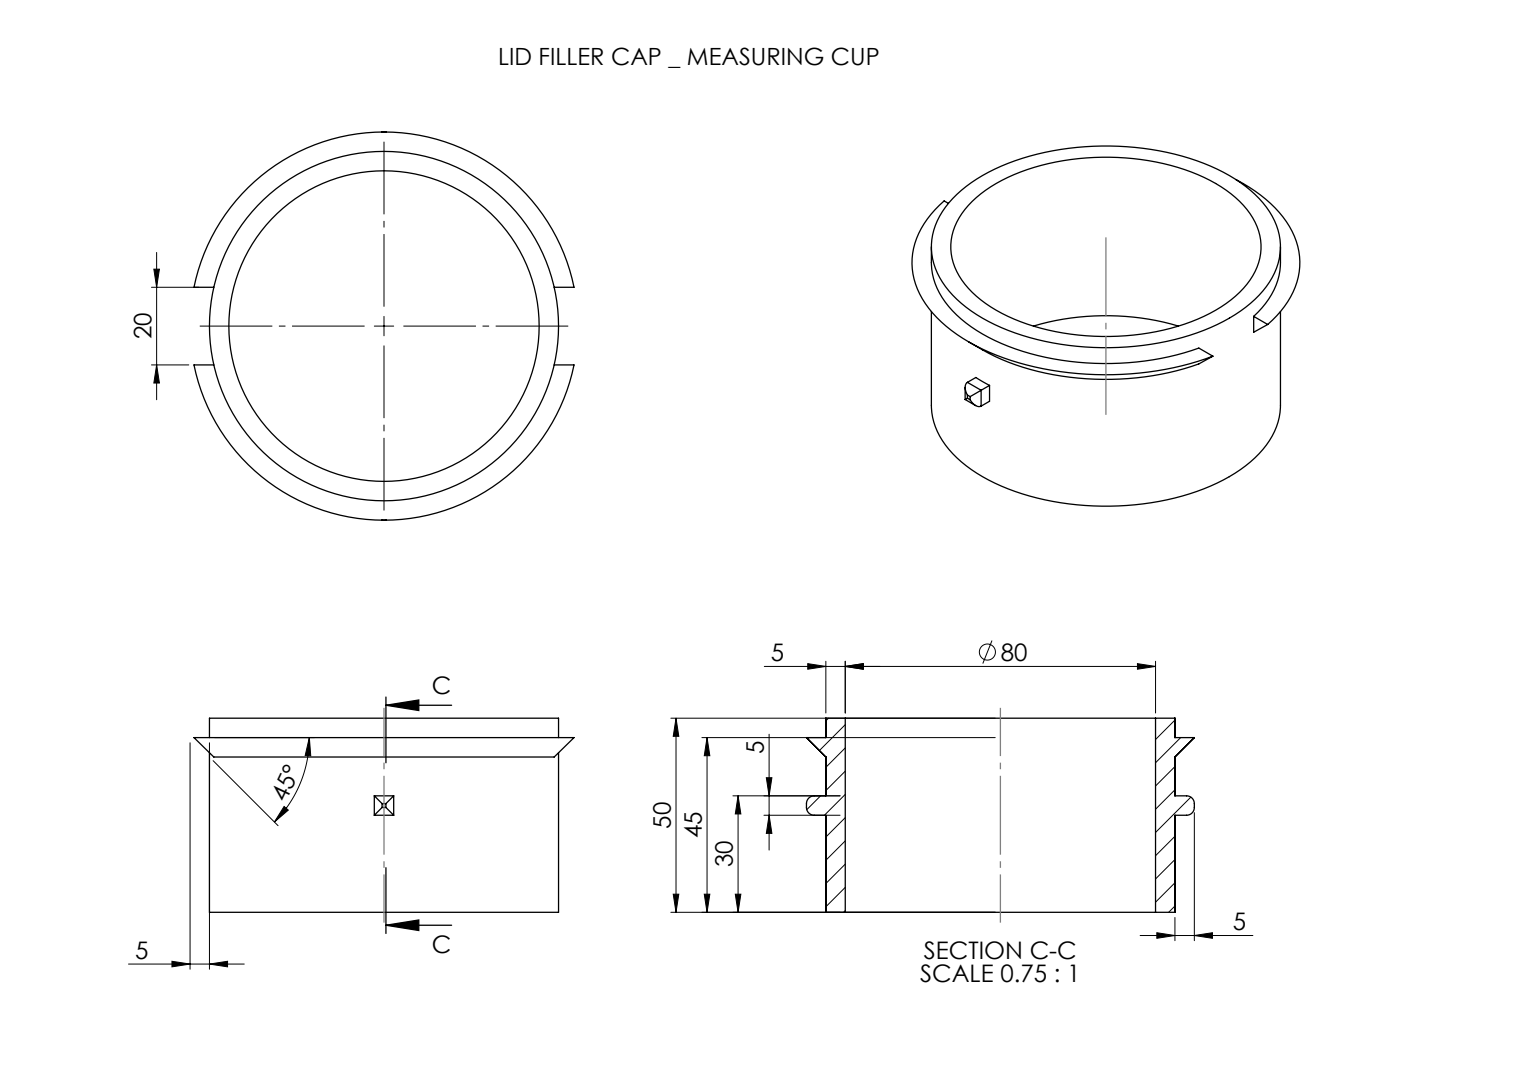
ISO-10303-21;
HEADER;
FILE_DESCRIPTION (('STEP AP214'),
    '1' );
FILE_NAME ('Lid Filler Cap _ Measuring Cup.step',
    '2026-10-09T15:02:13',
    ( '' ),
    ( '' ),
    'SwSTEP 2.0',
    'SolidWorks 2026',
    '' );
FILE_SCHEMA (( 'AUTOMOTIVE_DESIGN' ));
ENDSEC;

DATA;
#5=ORIENTED_EDGE ( 'NONE', *, *, #13422, .T. ) ;
#11=LINE ( 'NONE', #4013, #8670 ) ;
#38=CARTESIAN_POINT ( 'NONE',  ( -0.5000000000000000000, 247.0000000000000284, -49.99999999999999289 ) ) ;
#43=FACE_OUTER_BOUND ( 'NONE', #155, .T. ) ;
#49=( NAMED_UNIT ( * ) PLANE_ANGLE_UNIT ( ) SI_UNIT ( $, .RADIAN. ) );
#53=AXIS2_PLACEMENT_3D ( 'NONE', #15949, #12213, #9481 ) ;
#60=CARTESIAN_POINT ( 'NONE',  ( 48.98979485566356118, 261.9999999999999432, -10.00000000000000178 ) ) ;
#84=ADVANCED_FACE ( 'NONE', ( #9052 ), #9129, .T. ) ;
#99=EDGE_CURVE ( 'NONE', #10795, #16436, #8019, .T. ) ;
#105=CARTESIAN_POINT ( 'NONE',  ( 0.000000000000000000, 261.9999999999999432, 49.99999999999999289 ) ) ;
#115=CIRCLE ( 'NONE', #5192, 45.00000000000000000 ) ;
#121=AXIS2_PLACEMENT_3D ( 'NONE', #2630, #13768, #2460 ) ;
#129=( NAMED_UNIT ( * ) SI_UNIT ( $, .STERADIAN. ) SOLID_ANGLE_UNIT ( ) );
#140=AXIS2_PLACEMENT_3D ( 'NONE', #851, #930, #4703 ) ;
#149=LINE ( 'NONE', #6489, #8395 ) ;
#155=EDGE_LOOP ( 'NONE', ( #7318, #4198, #8287 ) ) ;
#161=PRESENTATION_STYLE_ASSIGNMENT (( #5178 ) ) ;
#164=CIRCLE ( 'NONE', #9467, 45.00000000000000000 ) ;
#227=DIRECTION ( 'NONE',  ( 0.000000000000000000, 0.000000000000000000, -1.000000000000000000 ) ) ;
#229=ORIENTED_EDGE ( 'NONE', *, *, #5927, .T. ) ;
#256=DIRECTION ( 'NONE',  ( 1.000000000000000000, -0.000000000000000000, 0.000000000000000000 ) ) ;
#260=CARTESIAN_POINT ( 'NONE',  ( 0.000000000000000000, 257.0000000000001137, 0.000000000000000000 ) ) ;
#277=LINE ( 'NONE', #1447, #969 ) ;
#314=DIRECTION ( 'NONE',  ( 0.000000000000000000, -1.000000000000000000, 0.000000000000000000 ) ) ;
#333=DIRECTION ( 'NONE',  ( 0.000000000000000000, 1.000000000000000000, 0.000000000000000000 ) ) ;
#350=DIRECTION ( 'NONE',  ( -0.000000000000000000, -1.000000000000000000, -0.000000000000000000 ) ) ;
#386=VECTOR ( 'NONE', #2589, 1000.000000000000000 ) ;
#407=EDGE_CURVE ( 'NONE', #5908, #14317, #4415, .T. ) ;
#409=CIRCLE ( 'NONE', #13951, 40.00000000000000000 ) ;
#441=EDGE_CURVE ( 'NONE', #7797, #13296, #9208, .T. ) ;
#442=AXIS2_PLACEMENT_3D ( 'NONE', #8820, #13970, #6598 ) ;
#469=ORIENTED_EDGE ( 'NONE', *, *, #407, .T. ) ;
#478=CARTESIAN_POINT ( 'NONE',  ( 0.5000000000000000000, 242.0000000000000284, -49.99999999999999289 ) ) ;
#516=CARTESIAN_POINT ( 'NONE',  ( 43.87482193696061472, 262.0000000000000000, -10.00000000000000000 ) ) ;
#573=CARTESIAN_POINT ( 'NONE',  ( 48.98979485566356118, 261.9999999999999432, -10.00000000000000178 ) ) ;
#590=EDGE_CURVE ( 'NONE', #9937, #12980, #2354, .T. ) ;
#613=ADVANCED_FACE ( 'NONE', ( #11344 ), #15222, .F. ) ;
#619=CIRCLE ( 'NONE', #8873, 45.00000000000000000 ) ;
#628=CARTESIAN_POINT ( 'NONE',  ( -43.87482193696060762, 257.0000000000001137, 10.00000000000000178 ) ) ;
#662=FACE_OUTER_BOUND ( 'NONE', #4298, .T. ) ;
#671=COLOUR_RGB ( '', 0.09019608, 0.27058824, 0.51372549) ;
#672=DIRECTION ( 'NONE',  ( 1.000000000000000000, 0.000000000000000000, -0.000000000000000000 ) ) ;
#693=VECTOR ( 'NONE', #7436, 1000.000000000000000 ) ;
#696=CIRCLE ( 'NONE', #10012, 45.00000000000000000 ) ;
#697=VECTOR ( 'NONE', #8943, 1000.000000000000000 ) ;
#709=AXIS2_PLACEMENT_3D ( 'NONE', #5217, #3952, #9026 ) ;
#716=EDGE_CURVE ( 'NONE', #9033, #5335, #1883, .T. ) ;
#740=ORIENTED_EDGE ( 'NONE', *, *, #6886, .T. ) ;
#751=CARTESIAN_POINT ( 'NONE',  ( -48.98979485566356828, 261.9999999999999432, -9.999999999999994671 ) ) ;
#799=ORIENTED_EDGE ( 'NONE', *, *, #441, .T. ) ;
#802=DIRECTION ( 'NONE',  ( 0.000000000000000000, 0.000000000000000000, 1.000000000000000000 ) ) ;
#814=ORIENTED_EDGE ( 'NONE', *, *, #8434, .F. ) ;
#826=EDGE_CURVE ( 'NONE', #11404, #10795, #164, .T. ) ;
#843=CARTESIAN_POINT ( 'NONE',  ( 0.000000000000000000, 267.0000000000000000, 0.000000000000000000 ) ) ;
#851=CARTESIAN_POINT ( 'NONE',  ( 0.000000000000000000, 247.0000000000000284, 0.000000000000000000 ) ) ;
#871=VERTEX_POINT ( 'NONE', #4096 ) ;
#930=DIRECTION ( 'NONE',  ( 0.000000000000000000, -1.000000000000000000, 0.000000000000000000 ) ) ;
#935=AXIS2_PLACEMENT_3D ( 'NONE', #14011, #3725, #13846 ) ;
#937=ORIENTED_EDGE ( 'NONE', *, *, #15743, .F. ) ;
#954=( GEOMETRIC_REPRESENTATION_CONTEXT ( 3 ) GLOBAL_UNCERTAINTY_ASSIGNED_CONTEXT ( ( #3259 ) ) GLOBAL_UNIT_ASSIGNED_CONTEXT ( ( #12888, #8987, #2830 ) ) REPRESENTATION_CONTEXT ( 'NONE', 'WORKASPACE' ) );
#958=DIRECTION ( 'NONE',  ( -0.000000000000000000, -1.000000000000000000, -0.000000000000000000 ) ) ;
#969=VECTOR ( 'NONE', #3869, 1000.000000000000000 ) ;
#1019=ADVANCED_FACE ( 'NONE', ( #14880 ), #4591, .T. ) ;
#1058=( BOUNDED_CURVE ( )  B_SPLINE_CURVE ( 3, ( #2059, #3401, #4566, #11138 ),
 .UNSPECIFIED., .F., .F. ) 
 B_SPLINE_CURVE_WITH_KNOTS ( ( 4, 4 ),
 ( 1.570796326794896780, 3.141592653589793116 ),
 .UNSPECIFIED. ) 
 CURVE ( )  GEOMETRIC_REPRESENTATION_ITEM ( )  RATIONAL_B_SPLINE_CURVE ( ( 1.000000000000000000, 0.8047378541243650485, 0.8047378541243650485, 1.000000000000000000 ) ) 
 REPRESENTATION_ITEM ( '' )  );
#1105=LINE ( 'NONE', #13997, #5701 ) ;
#1137=ORIENTED_EDGE ( 'NONE', *, *, #2862, .T. ) ;
#1152=DIRECTION ( 'NONE',  ( -0.000000000000000000, -1.000000000000000000, -0.000000000000000000 ) ) ;
#1159=VECTOR ( 'NONE', #14041, 1000.000000000000000 ) ;
#1167=DIRECTION ( 'NONE',  ( 0.000000000000000000, 0.000000000000000000, 1.000000000000000000 ) ) ;
#1174=CARTESIAN_POINT ( 'NONE',  ( 0.5000000000000000000, 244.0000000000000284, 49.99999999999999289 ) ) ;
#1176=DIRECTION ( 'NONE',  ( 1.000000000000000000, 0.000000000000000000, 0.000000000000000000 ) ) ;
#1191=DIRECTION ( 'NONE',  ( 1.000000000000000000, -0.000000000000000000, 0.000000000000000000 ) ) ;
#1216=( LENGTH_UNIT ( ) NAMED_UNIT ( * ) SI_UNIT ( .MILLI., .METRE. ) );
#1222=DIRECTION ( 'NONE',  ( -0.000000000000000000, 0.000000000000000000, -1.000000000000000000 ) ) ;
#1245=CARTESIAN_POINT ( 'NONE',  ( 2.500000000000000000, 242.0000000000000284, -47.99999999999999289 ) ) ;
#1256=DIRECTION ( 'NONE',  ( 0.000000000000000000, 0.000000000000000000, -1.000000000000000000 ) ) ;
#1301=FILL_AREA_STYLE ('',( #4995 ) ) ;
#1318=CARTESIAN_POINT ( 'NONE',  ( -2.500000000000000000, 242.0000000000000284, 40.00000000000000000 ) ) ;
#1323=ADVANCED_FACE ( 'NONE', ( #11720 ), #1654, .T. ) ;
#1328=VERTEX_POINT ( 'NONE', #9315 ) ;
#1335=PRODUCT_DEFINITION_SHAPE ( 'NONE', 'NONE',  #7215 ) ;
#1358=EDGE_CURVE ( 'NONE', #11111, #10385, #14441, .T. ) ;
#1359=DIRECTION ( 'NONE',  ( -0.000000000000000000, 1.000000000000000000, -0.000000000000000000 ) ) ;
#1364=PLANE ( 'NONE',  #709 ) ;
#1392=ORIENTED_EDGE ( 'NONE', *, *, #3028, .F. ) ;
#1394=CARTESIAN_POINT ( 'NONE',  ( 45.58196769024076644, 258.6644603543468861, -10.00000000000000178 ) ) ;
#1447=CARTESIAN_POINT ( 'NONE',  ( 0.000000000000000000, 242.0000000000000284, -47.99999999999999289 ) ) ;
#1454=CARTESIAN_POINT ( 'NONE',  ( -0.5000000000000000000, 244.0000000000000284, 49.99999999999999289 ) ) ;
#1465=ADVANCED_BREP_SHAPE_REPRESENTATION ( '', ( #14144, #15812 ), #5488 ) ;
#1490=CYLINDRICAL_SURFACE ( 'NONE', #7934, 40.00000000000000000 ) ;
#1491=CIRCLE ( 'NONE', #5765, 40.00000000000000000 ) ;
#1544=LINE ( 'NONE', #38, #15239 ) ;
#1555=CARTESIAN_POINT ( 'NONE',  ( 0.5000000000000000000, 245.0000000000000284, -49.99999999999999289 ) ) ;
#1581=ORIENTED_EDGE ( 'NONE', *, *, #8035, .T. ) ;
#1591=DIRECTION ( 'NONE',  ( 0.000000000000000000, -1.000000000000000000, 0.000000000000000000 ) ) ;
#1633=EDGE_CURVE ( 'NONE', #2064, #9033, #3918, .T. ) ;
#1645=LINE ( 'NONE', #10562, #16454 ) ;
#1654=CYLINDRICAL_SURFACE ( 'NONE', #4727, 2.000000000000001776 ) ;
#1661=ORIENTED_EDGE ( 'NONE', *, *, #2650, .F. ) ;
#1667=ORIENTED_EDGE ( 'NONE', *, *, #11380, .T. ) ;
#1686=DIRECTION ( 'NONE',  ( -1.000000000000000000, 0.000000000000000000, 0.000000000000000000 ) ) ;
#1700=VECTOR ( 'NONE', #10071, 1000.000000000000000 ) ;
#1704=EDGE_LOOP ( 'NONE', ( #4465, #8313, #12465, #9361 ) ) ;
#1759=CARTESIAN_POINT ( 'NONE',  ( -1.671572875253810153, 246.1715728752537871, -50.00000000000000000 ) ) ;
#1764=AXIS2_PLACEMENT_3D ( 'NONE', #2525, #15236, #15157 ) ;
#1805=ORIENTED_EDGE ( 'NONE', *, *, #3028, .T. ) ;
#1815=CARTESIAN_POINT ( 'NONE',  ( 0.000000000000000000, 242.0000000000000284, 0.000000000000000000 ) ) ;
#1825=CARTESIAN_POINT ( 'NONE',  ( -2.500000000000000000, 242.0000000000000284, -40.00000000000000000 ) ) ;
#1865=CARTESIAN_POINT ( 'NONE',  ( 0.000000000000000000, 217.0000000000000284, 0.000000000000000000 ) ) ;
#1883=( BOUNDED_CURVE ( )  B_SPLINE_CURVE ( 3, ( #11422, #10668, #1759, #14143 ),
 .UNSPECIFIED., .F., .F. ) 
 B_SPLINE_CURVE_WITH_KNOTS ( ( 4, 4 ),
 ( 3.141592653589793116, 4.712388980384689674 ),
 .UNSPECIFIED. ) 
 CURVE ( )  GEOMETRIC_REPRESENTATION_ITEM ( )  RATIONAL_B_SPLINE_CURVE ( ( 1.000000000000000000, 0.8047378541243649375, 0.8047378541243649375, 1.000000000000000000 ) ) 
 REPRESENTATION_ITEM ( '' )  );
#1911=CARTESIAN_POINT ( 'NONE',  ( 0.000000000000000000, 242.0000000000000284, 0.000000000000000000 ) ) ;
#1924=EDGE_CURVE ( 'NONE', #13942, #2064, #13776, .T. ) ;
#1931=DIRECTION ( 'NONE',  ( 0.000000000000000000, 1.000000000000000000, 0.000000000000000000 ) ) ;
#1943=CIRCLE ( 'NONE', #7794, 45.00000000000000000 ) ;
#1965=CARTESIAN_POINT ( 'NONE',  ( 0.000000000000000000, 261.9999999999999432, 0.000000000000000000 ) ) ;
#1968=CARTESIAN_POINT ( 'NONE',  ( 2.499999999999999556, 242.0000000000000284, -49.17157287525379417 ) ) ;
#1977=VERTEX_POINT ( 'NONE', #11381 ) ;
#1990=VECTOR ( 'NONE', #11855, 1000.000000000000000 ) ;
#2005=MECHANICAL_DESIGN_GEOMETRIC_PRESENTATION_REPRESENTATION('',(#13426),#15828);
#2028=MECHANICAL_DESIGN_GEOMETRIC_PRESENTATION_REPRESENTATION('',(#13447),#954);
#2054=CARTESIAN_POINT ( 'NONE',  ( -2.500000000000000000, 242.0000000000000284, 47.99999999999999289 ) ) ;
#2059=CARTESIAN_POINT ( 'NONE',  ( -0.5000000000000000000, 244.0000000000000284, 49.99999999999999289 ) ) ;
#2064=VERTEX_POINT ( 'NONE', #14677 ) ;
#2073=ORIENTED_EDGE ( 'NONE', *, *, #3686, .F. ) ;
#2110=ORIENTED_EDGE ( 'NONE', *, *, #14122, .T. ) ;
#2119=ORIENTED_EDGE ( 'NONE', *, *, #7947, .T. ) ;
#2122=ORIENTED_EDGE ( 'NONE', *, *, #13728, .T. ) ;
#2144=ORIENTED_EDGE ( 'NONE', *, *, #2862, .F. ) ;
#2154=CARTESIAN_POINT ( 'NONE',  ( -2.500000000000000000, 247.0000000000000284, 40.00000000000000000 ) ) ;
#2158=CARTESIAN_POINT ( 'NONE',  ( 0.000000000000000000, 0.000000000000000000, 0.000000000000000000 ) ) ;
#2161=DIRECTION ( 'NONE',  ( 0.000000000000000000, -1.000000000000000000, 0.000000000000000000 ) ) ;
#2189=AXIS2_PLACEMENT_3D ( 'NONE', #14664, #8362, #10630 ) ;
#2199=ORIENTED_EDGE ( 'NONE', *, *, #716, .T. ) ;
#2250=VERTEX_POINT ( 'NONE', #7390 ) ;
#2251=DIRECTION ( 'NONE',  ( -0.000000000000000000, -1.000000000000000000, -0.000000000000000000 ) ) ;
#2264=CARTESIAN_POINT ( 'NONE',  ( -0.5000000000000000000, 244.0000000000000284, -49.99999999999999289 ) ) ;
#2274=EDGE_CURVE ( 'NONE', #11502, #11404, #12970, .T. ) ;
#2295=EDGE_LOOP ( 'NONE', ( #3961, #2144 ) ) ;
#2305=CARTESIAN_POINT ( 'NONE',  ( 0.000000000000000000, 242.0000000000000284, 45.00000000000000000 ) ) ;
#2307=AXIS2_PLACEMENT_3D ( 'NONE', #15891, #14625, #3251 ) ;
#2308=CARTESIAN_POINT ( 'NONE',  ( 0.000000000000000000, 242.0000000000000284, 0.000000000000000000 ) ) ;
#2354=LINE ( 'NONE', #12578, #693 ) ;
#2380=FACE_OUTER_BOUND ( 'NONE', #2438, .T. ) ;
#2386=( LENGTH_UNIT ( ) NAMED_UNIT ( * ) SI_UNIT ( .MILLI., .METRE. ) );
#2408=CARTESIAN_POINT ( 'NONE',  ( -43.87482193696061472, 262.0000000000000000, 10.00000000000000178 ) ) ;
#2438=EDGE_LOOP ( 'NONE', ( #1392, #10459, #15571, #7122 ) ) ;
#2460=DIRECTION ( 'NONE',  ( 0.000000000000000000, 0.000000000000000000, 1.000000000000000000 ) ) ;
#2476=VERTEX_POINT ( 'NONE', #15965 ) ;
#2480=CARTESIAN_POINT ( 'NONE',  ( 4.898587196589413026E-15, 217.0000000000000284, -40.00000000000000000 ) ) ;
#2490=APPLICATION_CONTEXT ( 'automotive_design' ) ;
#2525=CARTESIAN_POINT ( 'NONE',  ( 0.000000000000000000, 262.0000000000000000, 0.000000000000000000 ) ) ;
#2530=DIRECTION ( 'NONE',  ( 0.000000000000000000, 0.000000000000000000, 1.000000000000000000 ) ) ;
#2565=ORIENTED_EDGE ( 'NONE', *, *, #99, .T. ) ;
#2570=AXIS2_PLACEMENT_3D ( 'NONE', #4839, #4664, #13620 ) ;
#2574=CARTESIAN_POINT ( 'NONE',  ( -43.87482193696061472, 257.0000000000001137, -10.00000000000000178 ) ) ;
#2589=DIRECTION ( 'NONE',  ( 1.000000000000000000, 0.000000000000000000, 0.000000000000000000 ) ) ;
#2600=DIRECTION ( 'NONE',  ( 0.000000000000000000, -1.000000000000000000, 0.000000000000000000 ) ) ;
#2626=ORIENTED_EDGE ( 'NONE', *, *, #7947, .F. ) ;
#2630=CARTESIAN_POINT ( 'NONE',  ( -0.5000000000000000000, 242.0000000000000284, 47.99999999999999289 ) ) ;
#2650=EDGE_CURVE ( 'NONE', #8967, #13787, #2656, .T. ) ;
#2653=CARTESIAN_POINT ( 'NONE',  ( 48.98979485566355407, 261.9999999999999432, 10.00000000000000178 ) ) ;
#2656=LINE ( 'NONE', #16381, #6623 ) ;
#2658=FACE_OUTER_BOUND ( 'NONE', #15932, .T. ) ;
#2661=ADVANCED_FACE ( 'NONE', ( #5016 ), #1490, .F. ) ;
#2673=DIRECTION ( 'NONE',  ( 0.000000000000000000, 0.000000000000000000, 1.000000000000000000 ) ) ;
#2688=ORIENTED_EDGE ( 'NONE', *, *, #3686, .T. ) ;
#2754=EDGE_CURVE ( 'NONE', #2831, #2833, #13123, .T. ) ;
#2773=CARTESIAN_POINT ( 'NONE',  ( 2.499999999999999556, 242.0000000000000284, 49.17157287525379417 ) ) ;
#2789=ORIENTED_EDGE ( 'NONE', *, *, #16426, .T. ) ;
#2801=CARTESIAN_POINT ( 'NONE',  ( 0.000000000000000000, 267.0000000000000000, 45.00000000000000000 ) ) ;
#2813=CARTESIAN_POINT ( 'NONE',  ( -2.500000000000000000, 242.0000000000000284, 40.00000000000000000 ) ) ;
#2817=AXIS2_PLACEMENT_3D ( 'NONE', #3359, #1931, #7024 ) ;
#2830=( NAMED_UNIT ( * ) SI_UNIT ( $, .STERADIAN. ) SOLID_ANGLE_UNIT ( ) );
#2831=VERTEX_POINT ( 'NONE', #4322 ) ;
#2833=VERTEX_POINT ( 'NONE', #2981 ) ;
#2862=EDGE_CURVE ( 'NONE', #8967, #11302, #6358, .T. ) ;
#2902=CARTESIAN_POINT ( 'NONE',  ( 0.000000000000000000, 257.0000000000001137, 0.000000000000000000 ) ) ;
#2918=ORIENTED_EDGE ( 'NONE', *, *, #4039, .T. ) ;
#2919=ORIENTED_EDGE ( 'NONE', *, *, #826, .T. ) ;
#2935=CYLINDRICAL_SURFACE ( 'NONE', #6732, 2.000000000000001776 ) ;
#2940=CARTESIAN_POINT ( 'NONE',  ( 2.500000000000000000, 242.0000000000000284, -49.99999999999999289 ) ) ;
#2959=DIRECTION ( 'NONE',  ( 0.000000000000000000, 0.000000000000000000, -1.000000000000000000 ) ) ;
#2960=CARTESIAN_POINT ( 'NONE',  ( -48.98979485566356118, 261.9999999999999432, 10.00000000000000178 ) ) ;
#2965=EDGE_CURVE ( 'NONE', #16436, #10385, #9551, .T. ) ;
#2981=CARTESIAN_POINT ( 'NONE',  ( -0.5000000000000000000, 245.0000000000000284, 49.99999999999999289 ) ) ;
#2990=CARTESIAN_POINT ( 'NONE',  ( -2.500000000000000000, 247.0000000000000284, -44.93050188902856945 ) ) ;
#3016=DIRECTION ( 'NONE',  ( -0.000000000000000000, -1.000000000000000000, -0.000000000000000000 ) ) ;
#3018=CARTESIAN_POINT ( 'NONE',  ( 0.5000000000000000000, 244.0000000000000284, 49.99999999999999289 ) ) ;
#3028=EDGE_CURVE ( 'NONE', #7197, #2833, #8692, .T. ) ;
#3031=VECTOR ( 'NONE', #12851, 1000.000000000000000 ) ;
#3035=CARTESIAN_POINT ( 'NONE',  ( -43.87482193696061472, 267.0000000000000000, -10.00000000000000178 ) ) ;
#3036=DIRECTION ( 'NONE',  ( -0.000000000000000000, 1.000000000000000000, -0.000000000000000000 ) ) ;
#3060=DIRECTION ( 'NONE',  ( -1.000000000000000000, -0.000000000000000000, -0.000000000000000000 ) ) ;
#3069=AXIS2_PLACEMENT_3D ( 'NONE', #3248, #6004, #16141 ) ;
#3076=VECTOR ( 'NONE', #2530, 1000.000000000000000 ) ;
#3157=VERTEX_POINT ( 'NONE', #2305 ) ;
#3183=CYLINDRICAL_SURFACE ( 'NONE', #4705, 2.000000000000001776 ) ;
#3239=DIRECTION ( 'NONE',  ( 1.000000000000000000, 0.000000000000000000, 0.000000000000000000 ) ) ;
#3248=CARTESIAN_POINT ( 'NONE',  ( 0.000000000000000000, 262.0000000000000000, 0.000000000000000000 ) ) ;
#3251=DIRECTION ( 'NONE',  ( 0.000000000000000000, 0.000000000000000000, 1.000000000000000000 ) ) ;
#3259=UNCERTAINTY_MEASURE_WITH_UNIT (LENGTH_MEASURE( 1.000000000000000082E-05 ), #12888, 'distance_accuracy_value', 'NONE');
#3309=DIRECTION ( 'NONE',  ( -0.000000000000000000, 1.000000000000000000, -0.000000000000000000 ) ) ;
#3322=FACE_OUTER_BOUND ( 'NONE', #12290, .T. ) ;
#3323=CARTESIAN_POINT ( 'NONE',  ( 0.000000000000000000, 217.0000000000000284, 0.000000000000000000 ) ) ;
#3325=LINE ( 'NONE', #5831, #7558 ) ;
#3341=ORIENTED_EDGE ( 'NONE', *, *, #9133, .T. ) ;
#3345=ORIENTED_EDGE ( 'NONE', *, *, #15831, .T. ) ;
#3347=CARTESIAN_POINT ( 'NONE',  ( 0.000000000000000000, 261.9999999999999432, 0.000000000000000000 ) ) ;
#3359=CARTESIAN_POINT ( 'NONE',  ( 0.000000000000000000, 257.0000000000001137, 0.000000000000000000 ) ) ;
#3373=EDGE_LOOP ( 'NONE', ( #1581, #13261, #7070, #7212 ) ) ;
#3400=CARTESIAN_POINT ( 'NONE',  ( -0.5000000000000000000, 245.0000000000000284, 49.99999999999999289 ) ) ;
#3401=CARTESIAN_POINT ( 'NONE',  ( -1.671572875253809487, 242.8284271247462129, 49.99999999999999289 ) ) ;
#3416=DIRECTION ( 'NONE',  ( -0.000000000000000000, 1.000000000000000000, -0.000000000000000000 ) ) ;
#3420=CARTESIAN_POINT ( 'NONE',  ( 2.500000000000000000, 247.0000000000000284, 47.99999999999999289 ) ) ;
#3427=CARTESIAN_POINT ( 'NONE',  ( 0.5000000000000000000, 245.0000000000000284, -49.99999999999999289 ) ) ;
#3456=VERTEX_POINT ( 'NONE', #2653 ) ;
#3471=ADVANCED_FACE ( 'NONE', ( #6329 ), #15195, .T. ) ;
#3487=DIRECTION ( 'NONE',  ( 1.000000000000000000, 0.000000000000000000, -0.000000000000000000 ) ) ;
#3496=CARTESIAN_POINT ( 'NONE',  ( 0.000000000000000000, 267.0000000000000000, 0.000000000000000000 ) ) ;
#3499=DIRECTION ( 'NONE',  ( -0.000000000000000000, -0.000000000000000000, -1.000000000000000000 ) ) ;
#3510=DIRECTION ( 'NONE',  ( 1.000000000000000000, 0.000000000000000000, 0.000000000000000000 ) ) ;
#3548=EDGE_LOOP ( 'NONE', ( #9663, #10724, #4831, #16342 ) ) ;
#3549=VECTOR ( 'NONE', #10900, 1000.000000000000000 ) ;
#3567=PLANE ( 'NONE',  #6457 ) ;
#3576=CYLINDRICAL_SURFACE ( 'NONE', #2570, 2.000000000000001776 ) ;
#3581=DIRECTION ( 'NONE',  ( 0.000000000000000000, 0.000000000000000000, 1.000000000000000000 ) ) ;
#3598=DIRECTION ( 'NONE',  ( 0.000000000000000000, -1.000000000000000000, 0.000000000000000000 ) ) ;
#3618=ORIENTED_EDGE ( 'NONE', *, *, #4491, .T. ) ;
#3625=CIRCLE ( 'NONE', #12915, 45.00000000000000000 ) ;
#3626=CIRCLE ( 'NONE', #5750, 45.00000000000000000 ) ;
#3684=ORIENTED_EDGE ( 'NONE', *, *, #7766, .F. ) ;
#3686=EDGE_CURVE ( 'NONE', #3456, #5700, #1645, .T. ) ;
#3687=EDGE_LOOP ( 'NONE', ( #8908, #8659, #937, #13226, #13943 ) ) ;
#3725=DIRECTION ( 'NONE',  ( 0.000000000000000000, 0.000000000000000000, -1.000000000000000000 ) ) ;
#3732=CARTESIAN_POINT ( 'NONE',  ( -2.500000000000000000, 242.0000000000000284, -40.00000000000000000 ) ) ;
#3758=VERTEX_POINT ( 'NONE', #4397 ) ;
#3781=ORIENTED_EDGE ( 'NONE', *, *, #8775, .T. ) ;
#3804=DIRECTION ( 'NONE',  ( 0.000000000000000000, 0.000000000000000000, -1.000000000000000000 ) ) ;
#3828=CARTESIAN_POINT ( 'NONE',  ( -45.00000000000000000, 262.0000000000000000, 10.00000000000000178 ) ) ;
#3829=DIRECTION ( 'NONE',  ( -0.000000000000000000, 1.000000000000000000, -0.000000000000000000 ) ) ;
#3830=CARTESIAN_POINT ( 'NONE',  ( 0.5000000000000000000, 247.0000000000000284, 49.99999999999999289 ) ) ;
#3839=CARTESIAN_POINT ( 'NONE',  ( 5.510910596163089556E-15, 217.0000000000000284, -45.00000000000000000 ) ) ;
#3869=DIRECTION ( 'NONE',  ( 1.000000000000000000, -0.000000000000000000, -0.000000000000000000 ) ) ;
#3878=ADVANCED_FACE ( 'NONE', ( #13205, #10801 ), #4318, .T. ) ;
#3883=PRODUCT_DEFINITION_FORMATION_WITH_SPECIFIED_SOURCE ( 'ANY', '', #8125, .NOT_KNOWN. ) ;
#3892=SURFACE_STYLE_FILL_AREA ( #1301 ) ;
#3896=AXIS2_PLACEMENT_3D ( 'NONE', #12478, #15963, #14700 ) ;
#3918=LINE ( 'NONE', #9070, #11352 ) ;
#3923=CARTESIAN_POINT ( 'NONE',  ( 45.58196769024076644, 258.6644603543468861, 10.00000000000000178 ) ) ;
#3927=CARTESIAN_POINT ( 'NONE',  ( 0.000000000000000000, 267.0000000000000000, 0.000000000000000000 ) ) ;
#3942=PRODUCT_DEFINITION_CONTEXT ( 'detailed design', #12378, 'design' ) ;
#3947=DIRECTION ( 'NONE',  ( 0.000000000000000000, 0.7071067811865362485, 0.7071067811865587860 ) ) ;
#3952=DIRECTION ( 'NONE',  ( -1.000000000000000000, 0.000000000000000000, 0.000000000000000000 ) ) ;
#3957=CARTESIAN_POINT ( 'NONE',  ( 2.500000000000000000, 245.0000000000000284, -49.99999999999999289 ) ) ;
#3961=ORIENTED_EDGE ( 'NONE', *, *, #4074, .F. ) ;
#4013=CARTESIAN_POINT ( 'NONE',  ( 0.000000000000000000, 247.0000000000000284, 47.99999999999999289 ) ) ;
#4039=EDGE_CURVE ( 'NONE', #16264, #14589, #15013, .T. ) ;
#4060=ADVANCED_FACE ( 'NONE', ( #15347 ), #12612, .T. ) ;
#4063=FACE_OUTER_BOUND ( 'NONE', #6879, .T. ) ;
#4073=DIRECTION ( 'NONE',  ( 0.000000000000000000, 0.000000000000000000, 1.000000000000000000 ) ) ;
#4074=EDGE_CURVE ( 'NONE', #11302, #8967, #409, .T. ) ;
#4094=CARTESIAN_POINT ( 'NONE',  ( -2.500000000000000000, 242.0000000000000284, 44.93050188902856945 ) ) ;
#4096=CARTESIAN_POINT ( 'NONE',  ( 2.500000000000000000, 242.0000000000000284, -44.93050188902856945 ) ) ;
#4163=VECTOR ( 'NONE', #3016, 1000.000000000000000 ) ;
#4170=CARTESIAN_POINT ( 'NONE',  ( 0.000000000000000000, 247.0000000000000284, 0.000000000000000000 ) ) ;
#4179=DIRECTION ( 'NONE',  ( -0.000000000000000000, -0.000000000000000000, -1.000000000000000000 ) ) ;
#4198=ORIENTED_EDGE ( 'NONE', *, *, #9133, .F. ) ;
#4221=FACE_OUTER_BOUND ( 'NONE', #8527, .T. ) ;
#4237=CARTESIAN_POINT ( 'NONE',  ( 0.5000000000000000000, 242.0000000000000284, 47.99999999999999289 ) ) ;
#4256=ORIENTED_EDGE ( 'NONE', *, *, #5027, .T. ) ;
#4258=DIRECTION ( 'NONE',  ( 1.000000000000000000, 0.000000000000000000, 0.000000000000000000 ) ) ;
#4280=CARTESIAN_POINT ( 'NONE',  ( 2.500000000000000000, 242.0000000000000284, 47.99999999999999289 ) ) ;
#4294=CARTESIAN_POINT ( 'NONE',  ( 2.500000000000000000, 244.0000000000000284, -49.99999999999999289 ) ) ;
#4298=EDGE_LOOP ( 'NONE', ( #16151, #2919, #2565, #11055, #3341 ) ) ;
#4301=ADVANCED_FACE ( 'NONE', ( #4221 ), #9288, .T. ) ;
#4312=VERTEX_POINT ( 'NONE', #2960 ) ;
#4315=DIRECTION ( 'NONE',  ( 0.000000000000000000, 0.000000000000000000, -1.000000000000000000 ) ) ;
#4318=PLANE ( 'NONE',  #14478 ) ;
#4322=CARTESIAN_POINT ( 'NONE',  ( 0.5000000000000000000, 245.0000000000000284, 49.99999999999999289 ) ) ;
#4324=DIRECTION ( 'NONE',  ( 0.000000000000000000, -1.000000000000000000, 0.000000000000000000 ) ) ;
#4326=DIRECTION ( 'NONE',  ( -1.000000000000000000, 0.000000000000000000, 0.000000000000000000 ) ) ;
#4329=CARTESIAN_POINT ( 'NONE',  ( 43.87482193696061472, 257.0000000000001137, 10.00000000000000178 ) ) ;
#4339=AXIS2_PLACEMENT_3D ( 'NONE', #12987, #1591, #6685 ) ;
#4358=CARTESIAN_POINT ( 'NONE',  ( -47.28673853953970507, 260.3313524089090265, 10.00000000000000178 ) ) ;
#4361=VECTOR ( 'NONE', #1152, 1000.000000000000000 ) ;
#4392=ORIENTED_EDGE ( 'NONE', *, *, #8165, .T. ) ;
#4393=ORIENTED_EDGE ( 'NONE', *, *, #2274, .F. ) ;
#4397=CARTESIAN_POINT ( 'NONE',  ( 5.510910596163089556E-15, 247.0000000000000284, -45.00000000000000000 ) ) ;
#4415=CIRCLE ( 'NONE', #2817, 45.00000000000000000 ) ;
#4437=AXIS2_PLACEMENT_3D ( 'NONE', #2308, #9629, #15018 ) ;
#4448=VECTOR ( 'NONE', #1191, 1000.000000000000000 ) ;
#4462=EDGE_LOOP ( 'NONE', ( #2789, #14991, #12051, #16393, #13020, #2688 ) ) ;
#4465=ORIENTED_EDGE ( 'NONE', *, *, #7682, .T. ) ;
#4481=ORIENTED_EDGE ( 'NONE', *, *, #15955, .F. ) ;
#4491=EDGE_CURVE ( 'NONE', #12980, #7494, #8769, .T. ) ;
#4496=ORIENTED_EDGE ( 'NONE', *, *, #16426, .F. ) ;
#4518=AXIS2_PLACEMENT_3D ( 'NONE', #1965, #5812, #4565 ) ;
#4530=CYLINDRICAL_SURFACE ( 'NONE', #7074, 2.000000000000001776 ) ;
#4565=DIRECTION ( 'NONE',  ( 0.000000000000000000, 0.000000000000000000, -1.000000000000000000 ) ) ;
#4566=CARTESIAN_POINT ( 'NONE',  ( -2.499999999999999556, 242.0000000000000284, 49.17157287525379417 ) ) ;
#4583=FACE_OUTER_BOUND ( 'NONE', #6617, .T. ) ;
#4591=PLANE ( 'NONE',  #10558 ) ;
#4597=CARTESIAN_POINT ( 'NONE',  ( -2.500000000000000000, 217.0000000000000284, -44.93050188902856945 ) ) ;
#4635=PLANE ( 'NONE',  #2189 ) ;
#4662=ORIENTED_EDGE ( 'NONE', *, *, #8269, .F. ) ;
#4664=DIRECTION ( 'NONE',  ( 0.000000000000000000, 1.000000000000000000, 0.000000000000000000 ) ) ;
#4673=VECTOR ( 'NONE', #5576, 1000.000000000000000 ) ;
#4698=CLOSED_SHELL ( 'NONE', ( #6928, #10284, #4060, #14884, #6739, #4301, #3878, #8847, #2661, #10035, #10518, #14607, #11167, #11202, #1019, #613, #6021, #12253, #3471, #13850, #5707, #11911, #1323, #84, #15145, #9635, #11125, #4837, #12291, #9610, #10662, #9826, #11496 ) ) ;
#4703=DIRECTION ( 'NONE',  ( 0.000000000000000000, 0.000000000000000000, -1.000000000000000000 ) ) ;
#4705=AXIS2_PLACEMENT_3D ( 'NONE', #15903, #10676, #15575 ) ;
#4727=AXIS2_PLACEMENT_3D ( 'NONE', #11884, #4326, #4073 ) ;
#4756=ORIENTED_EDGE ( 'NONE', *, *, #15914, .F. ) ;
#4774=DIRECTION ( 'NONE',  ( 0.000000000000000000, 0.000000000000000000, 1.000000000000000000 ) ) ;
#4799=ORIENTED_EDGE ( 'NONE', *, *, #9262, .F. ) ;
#4802=ORIENTED_EDGE ( 'NONE', *, *, #14156, .F. ) ;
#4831=ORIENTED_EDGE ( 'NONE', *, *, #1924, .F. ) ;
#4837=ADVANCED_FACE ( 'NONE', ( #15906 ), #4530, .T. ) ;
#4839=CARTESIAN_POINT ( 'NONE',  ( 0.5000000000000000000, 242.0000000000000284, -47.99999999999999289 ) ) ;
#4909=SHAPE_REPRESENTATION_RELATIONSHIP ( 'NONE' , 'NONE' ,  #5560, #1465 ) ;
#4933=DIRECTION ( 'NONE',  ( 0.000000000000000000, 0.000000000000000000, 1.000000000000000000 ) ) ;
#4936=AXIS2_PLACEMENT_3D ( 'NONE', #13137, #15707, #4258 ) ;
#4943=ORIENTED_EDGE ( 'NONE', *, *, #5027, .F. ) ;
#4965=EDGE_LOOP ( 'NONE', ( #740, #12195, #4756 ) ) ;
#4995=FILL_AREA_STYLE_COLOUR ( '', #671 ) ;
#5015=LINE ( 'NONE', #1318, #7534 ) ;
#5016=FACE_OUTER_BOUND ( 'NONE', #5518, .T. ) ;
#5027=EDGE_CURVE ( 'NONE', #7197, #7494, #11, .T. ) ;
#5042=CARTESIAN_POINT ( 'NONE',  ( 0.000000000000000000, 247.0000000000000284, 0.000000000000000000 ) ) ;
#5089=CARTESIAN_POINT ( 'NONE',  ( -2.500000000000000000, 242.0000000000000284, 49.99999999999999289 ) ) ;
#5092=DIRECTION ( 'NONE',  ( 0.000000000000000000, 0.000000000000000000, 1.000000000000000000 ) ) ;
#5095=LINE ( 'NONE', #15200, #4361 ) ;
#5157=EDGE_LOOP ( 'NONE', ( #8102, #10104, #5992, #5888 ) ) ;
#5165=CARTESIAN_POINT ( 'NONE',  ( 47.28673853953970507, 260.3313524089090265, -10.00000000000000178 ) ) ;
#5172=CARTESIAN_POINT ( 'NONE',  ( 0.000000000000000000, 217.0000000000000284, 0.000000000000000000 ) ) ;
#5178=SURFACE_STYLE_USAGE ( .BOTH. , #7737 ) ;
#5183=LINE ( 'NONE', #8993, #386 ) ;
#5192=AXIS2_PLACEMENT_3D ( 'NONE', #3323, #14950, #3239 ) ;
#5217=CARTESIAN_POINT ( 'NONE',  ( 2.500000000000000000, 242.0000000000000284, 40.00000000000000000 ) ) ;
#5223=( BOUNDED_CURVE ( )  B_SPLINE_CURVE ( 3, ( #13453, #12036, #1968, #9557 ),
 .UNSPECIFIED., .F., .T. ) 
 B_SPLINE_CURVE_WITH_KNOTS ( ( 4, 4 ),
 ( 1.570796326794896780, 3.141592653589793116 ),
 .UNSPECIFIED. ) 
 CURVE ( )  GEOMETRIC_REPRESENTATION_ITEM ( )  RATIONAL_B_SPLINE_CURVE ( ( 1.000000000000000000, 0.8047378541243650485, 0.8047378541243650485, 1.000000000000000000 ) ) 
 REPRESENTATION_ITEM ( '' )  );
#5228=EDGE_LOOP ( 'NONE', ( #799, #9813, #2199, #4662 ) ) ;
#5237=DIRECTION ( 'NONE',  ( -0.000000000000000000, 1.000000000000000000, -0.000000000000000000 ) ) ;
#5295=ORIENTED_EDGE ( 'NONE', *, *, #10543, .T. ) ;
#5335=VERTEX_POINT ( 'NONE', #8809 ) ;
#5357=CARTESIAN_POINT ( 'NONE',  ( 0.000000000000000000, 267.0000000000000000, 0.000000000000000000 ) ) ;
#5413=CARTESIAN_POINT ( 'NONE',  ( -2.500000000000000000, 245.0000000000000284, 49.99999999999999289 ) ) ;
#5421=DIRECTION ( 'NONE',  ( 0.000000000000000000, 0.000000000000000000, -1.000000000000000000 ) ) ;
#5449=FACE_OUTER_BOUND ( 'NONE', #5157, .T. ) ;
#5468=VERTEX_POINT ( 'NONE', #2408 ) ;
#5488=( GEOMETRIC_REPRESENTATION_CONTEXT ( 3 ) GLOBAL_UNCERTAINTY_ASSIGNED_CONTEXT ( ( #12067 ) ) GLOBAL_UNIT_ASSIGNED_CONTEXT ( ( #2386, #13690, #16444 ) ) REPRESENTATION_CONTEXT ( 'NONE', 'WORKASPACE' ) );
#5498=CIRCLE ( 'NONE', #14753, 40.00000000000000000 ) ;
#5518=EDGE_LOOP ( 'NONE', ( #1661, #1137, #2119, #5851 ) ) ;
#5529=AXIS2_PLACEMENT_3D ( 'NONE', #2813, #5575, #11635 ) ;
#5540=LINE ( 'NONE', #4280, #4163 ) ;
#5560=SHAPE_REPRESENTATION ( 'Lid Filler Cap _ Measuring Cup', ( #15812 ), #5488 ) ;
#5564=DIRECTION ( 'NONE',  ( -1.000000000000000000, 0.000000000000000000, 0.000000000000000000 ) ) ;
#5575=DIRECTION ( 'NONE',  ( -1.000000000000000000, 0.000000000000000000, 0.000000000000000000 ) ) ;
#5576=DIRECTION ( 'NONE',  ( -0.000000000000000000, -1.000000000000000000, -0.000000000000000000 ) ) ;
#5577=DIRECTION ( 'NONE',  ( 0.000000000000000000, -0.000000000000000000, -1.000000000000000000 ) ) ;
#5643=FACE_OUTER_BOUND ( 'NONE', #3373, .T. ) ;
#5700=VERTEX_POINT ( 'NONE', #10781 ) ;
#5701=VECTOR ( 'NONE', #1359, 1000.000000000000000 ) ;
#5702=DIRECTION ( 'NONE',  ( -1.000000000000000000, 0.000000000000000000, 0.000000000000000000 ) ) ;
#5707=ADVANCED_FACE ( 'NONE', ( #6725 ), #10545, .T. ) ;
#5721=ORIENTED_EDGE ( 'NONE', *, *, #2754, .T. ) ;
#5725=CARTESIAN_POINT ( 'NONE',  ( 2.500000000000000000, 242.0000000000000284, -47.99999999999999289 ) ) ;
#5750=AXIS2_PLACEMENT_3D ( 'NONE', #14715, #8498, #6104 ) ;
#5753=CARTESIAN_POINT ( 'NONE',  ( -2.500000000000000000, 242.0000000000000284, -47.99999999999999289 ) ) ;
#5765=AXIS2_PLACEMENT_3D ( 'NONE', #843, #3598, #10002 ) ;
#5773=VECTOR ( 'NONE', #14163, 1000.000000000000000 ) ;
#5807=DIRECTION ( 'NONE',  ( -1.000000000000000000, 0.000000000000000000, 0.000000000000000000 ) ) ;
#5812=DIRECTION ( 'NONE',  ( -0.000000000000000000, -1.000000000000000000, -0.000000000000000000 ) ) ;
#5815=CARTESIAN_POINT ( 'NONE',  ( -2.500000000000000000, 247.0000000000000284, 47.99999999999999289 ) ) ;
#5831=CARTESIAN_POINT ( 'NONE',  ( 0.000000000000000000, 217.0000000000000284, 40.00000000000000000 ) ) ;
#5834=CARTESIAN_POINT ( 'NONE',  ( 0.000000000000000000, 261.9999999999999432, 0.000000000000000000 ) ) ;
#5835=LINE ( 'NONE', #8239, #3549 ) ;
#5851=ORIENTED_EDGE ( 'NONE', *, *, #13222, .F. ) ;
#5886=EDGE_LOOP ( 'NONE', ( #10870, #11725, #2073 ) ) ;
#5888=ORIENTED_EDGE ( 'NONE', *, *, #5959, .F. ) ;
#5908=VERTEX_POINT ( 'NONE', #7772 ) ;
#5916=EDGE_CURVE ( 'NONE', #13296, #9545, #277, .T. ) ;
#5927=EDGE_CURVE ( 'NONE', #2250, #10795, #10192, .T. ) ;
#5959=EDGE_CURVE ( 'NONE', #8386, #6499, #10353, .T. ) ;
#5978=CARTESIAN_POINT ( 'NONE',  ( -1.671572875253810153, 246.1715728752537871, 50.00000000000000000 ) ) ;
#5987=EDGE_CURVE ( 'NONE', #3758, #11404, #11514, .T. ) ;
#5992=ORIENTED_EDGE ( 'NONE', *, *, #8035, .F. ) ;
#6000=CARTESIAN_POINT ( 'NONE',  ( 0.000000000000000000, 267.0000000000000000, 0.000000000000000000 ) ) ;
#6004=DIRECTION ( 'NONE',  ( -0.000000000000000000, -1.000000000000000000, -0.000000000000000000 ) ) ;
#6013=ORIENTED_EDGE ( 'NONE', *, *, #441, .F. ) ;
#6017=ORIENTED_EDGE ( 'NONE', *, *, #13167, .F. ) ;
#6021=ADVANCED_FACE ( 'NONE', ( #12765 ), #1364, .F. ) ;
#6030=AXIS2_PLACEMENT_3D ( 'NONE', #6699, #672, #13081 ) ;
#6089=CARTESIAN_POINT ( 'NONE',  ( 0.5000000000000000000, 245.0000000000000284, 49.99999999999999289 ) ) ;
#6099=DIRECTION ( 'NONE',  ( 0.000000000000000000, 1.000000000000000000, 0.000000000000000000 ) ) ;
#6104=DIRECTION ( 'NONE',  ( 0.000000000000000000, 0.000000000000000000, -1.000000000000000000 ) ) ;
#6136=ORIENTED_EDGE ( 'NONE', *, *, #11659, .F. ) ;
#6181=FACE_OUTER_BOUND ( 'NONE', #4462, .T. ) ;
#6218=EDGE_CURVE ( 'NONE', #14271, #3758, #11571, .T. ) ;
#6223=AXIS2_PLACEMENT_3D ( 'NONE', #8810, #10148, #4933 ) ;
#6233=VECTOR ( 'NONE', #3499, 1000.000000000000000 ) ;
#6259=CARTESIAN_POINT ( 'NONE',  ( 48.98979485566355407, 261.9999999999999432, 10.00000000000000178 ) ) ;
#6280=ORIENTED_EDGE ( 'NONE', *, *, #11036, .F. ) ;
#6305=CARTESIAN_POINT ( 'NONE',  ( 0.000000000000000000, 217.0000000000000284, 0.000000000000000000 ) ) ;
#6329=FACE_OUTER_BOUND ( 'NONE', #10890, .T. ) ;
#6348=CARTESIAN_POINT ( 'NONE',  ( 0.000000000000000000, 217.0000000000000284, 0.000000000000000000 ) ) ;
#6358=CIRCLE ( 'NONE', #15633, 40.00000000000000000 ) ;
#6392=SURFACE_SIDE_STYLE ('',( #3892 ) ) ;
#6415=CARTESIAN_POINT ( 'NONE',  ( 0.000000000000000000, 242.0000000000000284, 0.000000000000000000 ) ) ;
#6452=CARTESIAN_POINT ( 'NONE',  ( 2.500000000000000000, 247.0000000000000284, 40.00000000000000000 ) ) ;
#6457=AXIS2_PLACEMENT_3D ( 'NONE', #3732, #3487, #1222 ) ;
#6479=DIRECTION ( 'NONE',  ( 1.000000000000000000, 0.000000000000000000, 0.000000000000000000 ) ) ;
#6487=DIRECTION ( 'NONE',  ( -0.000000000000000000, 0.000000000000000000, 1.000000000000000000 ) ) ;
#6489=CARTESIAN_POINT ( 'NONE',  ( -2.500000000000000000, 242.0000000000000284, -47.99999999999999289 ) ) ;
#6499=VERTEX_POINT ( 'NONE', #1174 ) ;
#6521=B_SPLINE_CURVE_WITH_KNOTS ( 'NONE', 3,
 ( #60, #5165, #1394, #15275 ),
 .UNSPECIFIED., .F., .F.,
 ( 4, 4 ),
 ( 0.01002676606614814371, 0.01717959331248046853 ),
 .UNSPECIFIED. ) ;
#6523=AXIS2_PLACEMENT_3D ( 'NONE', #3035, #2959, #8106 ) ;
#6571=VERTEX_POINT ( 'NONE', #4094 ) ;
#6572=CARTESIAN_POINT ( 'NONE',  ( -47.28673853953969797, 260.3313524089090265, -10.00000000000000178 ) ) ;
#6589=DIRECTION ( 'NONE',  ( 1.000000000000000000, 0.000000000000000000, 0.000000000000000000 ) ) ;
#6592=DIRECTION ( 'NONE',  ( 0.000000000000000000, -1.000000000000000000, 0.000000000000000000 ) ) ;
#6598=DIRECTION ( 'NONE',  ( 1.000000000000000000, 0.000000000000000000, -0.000000000000000000 ) ) ;
#6601=DIRECTION ( 'NONE',  ( -0.000000000000000000, 1.000000000000000000, -0.000000000000000000 ) ) ;
#6617=EDGE_LOOP ( 'NONE', ( #3684, #469, #9794, #12943 ) ) ;
#6618=LINE ( 'NONE', #7604, #7345 ) ;
#6623=VECTOR ( 'NONE', #12881, 1000.000000000000000 ) ;
#6657=VERTEX_POINT ( 'NONE', #3427 ) ;
#6660=LINE ( 'NONE', #14280, #4673 ) ;
#6683=DIRECTION ( 'NONE',  ( -0.000000000000000000, 1.000000000000000000, -0.000000000000000000 ) ) ;
#6685=DIRECTION ( 'NONE',  ( 0.000000000000000000, 0.000000000000000000, -1.000000000000000000 ) ) ;
#6696=ORIENTED_EDGE ( 'NONE', *, *, #4491, .F. ) ;
#6699=CARTESIAN_POINT ( 'NONE',  ( 2.500000000000000000, 242.0000000000000284, -40.00000000000000000 ) ) ;
#6716=ORIENTED_EDGE ( 'NONE', *, *, #14306, .T. ) ;
#6718=LINE ( 'NONE', #7950, #1990 ) ;
#6725=FACE_OUTER_BOUND ( 'NONE', #10344, .T. ) ;
#6727=PRODUCT_CONTEXT ( 'NONE', #2490, 'mechanical' ) ;
#6732=AXIS2_PLACEMENT_3D ( 'NONE', #8002, #13076, #10594 ) ;
#6739=ADVANCED_FACE ( 'NONE', ( #662 ), #14593, .T. ) ;
#6785=VECTOR ( 'NONE', #3416, 1000.000000000000000 ) ;
#6809=SHAPE_DEFINITION_REPRESENTATION ( #1335, #5560 ) ;
#6825=AXIS2_PLACEMENT_3D ( 'NONE', #12870, #6479, #227 ) ;
#6861=DIRECTION ( 'NONE',  ( 0.000000000000000000, 0.000000000000000000, 1.000000000000000000 ) ) ;
#6879=EDGE_LOOP ( 'NONE', ( #15611, #14191, #13747, #11446 ) ) ;
#6886=EDGE_CURVE ( 'NONE', #5468, #9544, #5095, .T. ) ;
#6907=DIRECTION ( 'NONE',  ( 0.000000000000000000, 0.000000000000000000, -1.000000000000000000 ) ) ;
#6912=ORIENTED_EDGE ( 'NONE', *, *, #8796, .T. ) ;
#6913=( BOUNDED_CURVE ( )  B_SPLINE_CURVE ( 3, ( #3018, #13163, #2773, #10516 ),
 .UNSPECIFIED., .F., .F. ) 
 B_SPLINE_CURVE_WITH_KNOTS ( ( 4, 4 ),
 ( 1.570796326794896780, 3.141592653589793116 ),
 .UNSPECIFIED. ) 
 CURVE ( )  GEOMETRIC_REPRESENTATION_ITEM ( )  RATIONAL_B_SPLINE_CURVE ( ( 1.000000000000000000, 0.8047378541243650485, 0.8047378541243650485, 1.000000000000000000 ) ) 
 REPRESENTATION_ITEM ( '' )  );
#6928=ADVANCED_FACE ( 'NONE', ( #2658 ), #10467, .T. ) ;
#6936=EDGE_CURVE ( 'NONE', #6499, #2831, #7567, .T. ) ;
#6940=CARTESIAN_POINT ( 'NONE',  ( -48.98979485566356118, 261.9999999999999432, 10.00000000000000178 ) ) ;
#6967=EDGE_CURVE ( 'NONE', #14589, #7197, #13715, .T. ) ;
#6979=DIRECTION ( 'NONE',  ( -0.000000000000000000, -1.000000000000000000, -0.000000000000000000 ) ) ;
#6985=ORIENTED_EDGE ( 'NONE', *, *, #15743, .T. ) ;
#7010=LINE ( 'NONE', #4597, #10703 ) ;
#7015=DIRECTION ( 'NONE',  ( -0.000000000000000000, 0.000000000000000000, -1.000000000000000000 ) ) ;
#7024=DIRECTION ( 'NONE',  ( 0.000000000000000000, 0.000000000000000000, 1.000000000000000000 ) ) ;
#7041=CIRCLE ( 'NONE', #4936, 45.00000000000000000 ) ;
#7058=EDGE_CURVE ( 'NONE', #2476, #871, #619, .T. ) ;
#7063=VECTOR ( 'NONE', #14789, 1000.000000000000000 ) ;
#7070=ORIENTED_EDGE ( 'NONE', *, *, #10581, .T. ) ;
#7074=AXIS2_PLACEMENT_3D ( 'NONE', #9593, #14640, #9764 ) ;
#7075=AXIS2_PLACEMENT_3D ( 'NONE', #15062, #9668, #14808 ) ;
#7083=LINE ( 'NONE', #7327, #11315 ) ;
#7084=DIRECTION ( 'NONE',  ( 0.000000000000000000, -1.000000000000000000, 0.000000000000000000 ) ) ;
#7122=ORIENTED_EDGE ( 'NONE', *, *, #9357, .F. ) ;
#7154=EDGE_LOOP ( 'NONE', ( #1667, #9461 ) ) ;
#7163=ORIENTED_EDGE ( 'NONE', *, *, #7330, .F. ) ;
#7182=CARTESIAN_POINT ( 'NONE',  ( 2.500000000000000000, 247.0000000000000284, 44.93050188902856945 ) ) ;
#7197=VERTEX_POINT ( 'NONE', #5815 ) ;
#7212=ORIENTED_EDGE ( 'NONE', *, *, #6936, .F. ) ;
#7215=PRODUCT_DEFINITION ( 'UNKNOWN', '', #3883, #3942 ) ;
#7237=DIRECTION ( 'NONE',  ( 0.000000000000000000, -0.000000000000000000, -1.000000000000000000 ) ) ;
#7244=LINE ( 'NONE', #8317, #8862 ) ;
#7274=CARTESIAN_POINT ( 'NONE',  ( -1.671572875253809487, 242.8284271247462129, -50.00000000000000000 ) ) ;
#7304=VECTOR ( 'NONE', #4179, 1000.000000000000000 ) ;
#7318=ORIENTED_EDGE ( 'NONE', *, *, #11093, .T. ) ;
#7327=CARTESIAN_POINT ( 'NONE',  ( -2.500000000000000000, 217.0000000000000284, 44.93050188902856945 ) ) ;
#7330=EDGE_CURVE ( 'NONE', #9682, #9545, #5223, .T. ) ;
#7345=VECTOR ( 'NONE', #350, 1000.000000000000000 ) ;
#7358=AXIS2_PLACEMENT_3D ( 'NONE', #4170, #6592, #5421 ) ;
#7368=VECTOR ( 'NONE', #6589, 1000.000000000000000 ) ;
#7390=CARTESIAN_POINT ( 'NONE',  ( -43.87482193696061472, 262.0000000000000000, -10.00000000000000178 ) ) ;
#7421=ORIENTED_EDGE ( 'NONE', *, *, #11209, .T. ) ;
#7426=DIRECTION ( 'NONE',  ( 0.000000000000000000, 1.000000000000000000, 0.000000000000000000 ) ) ;
#7436=DIRECTION ( 'NONE',  ( -0.000000000000000000, 1.000000000000000000, -0.000000000000000000 ) ) ;
#7494=VERTEX_POINT ( 'NONE', #8964 ) ;
#7500=DIRECTION ( 'NONE',  ( 0.000000000000000000, -1.000000000000000000, -0.000000000000000000 ) ) ;
#7534=VECTOR ( 'NONE', #5092, 1000.000000000000000 ) ;
#7556=ORIENTED_EDGE ( 'NONE', *, *, #13811, .F. ) ;
#7558=VECTOR ( 'NONE', #10603, 1000.000000000000000 ) ;
#7567=LINE ( 'NONE', #3830, #1159 ) ;
#7582=CYLINDRICAL_SURFACE ( 'NONE', #8122, 40.00000000000000000 ) ;
#7593=AXIS2_PLACEMENT_3D ( 'NONE', #11374, #5237, #7706 ) ;
#7604=CARTESIAN_POINT ( 'NONE',  ( 43.87482193696061472, 267.0000000000000000, -10.00000000000000000 ) ) ;
#7621=LINE ( 'NONE', #3957, #3031 ) ;
#7640=VERTEX_POINT ( 'NONE', #14268 ) ;
#7682=EDGE_CURVE ( 'NONE', #2064, #6657, #13684, .T. ) ;
#7706=DIRECTION ( 'NONE',  ( 0.000000000000000000, 0.000000000000000000, 1.000000000000000000 ) ) ;
#7715=ORIENTED_EDGE ( 'NONE', *, *, #7682, .F. ) ;
#7718=ORIENTED_EDGE ( 'NONE', *, *, #11659, .T. ) ;
#7722=ORIENTED_EDGE ( 'NONE', *, *, #6936, .T. ) ;
#7737=SURFACE_SIDE_STYLE ('',( #15293 ) ) ;
#7742=DIRECTION ( 'NONE',  ( 0.000000000000000000, 0.000000000000000000, 1.000000000000000000 ) ) ;
#7766=EDGE_CURVE ( 'NONE', #5908, #1328, #10029, .T. ) ;
#7772=CARTESIAN_POINT ( 'NONE',  ( 0.000000000000000000, 257.0000000000001137, 45.00000000000000000 ) ) ;
#7778=EDGE_CURVE ( 'NONE', #871, #13942, #1105, .T. ) ;
#7794=AXIS2_PLACEMENT_3D ( 'NONE', #6000, #7084, #11070 ) ;
#7797=VERTEX_POINT ( 'NONE', #12592 ) ;
#7821=PLANE ( 'NONE',  #442 ) ;
#7844=ORIENTED_EDGE ( 'NONE', *, *, #7330, .T. ) ;
#7875=CARTESIAN_POINT ( 'NONE',  ( 1.671572875253809487, 246.1715728752537871, -50.00000000000000000 ) ) ;
#7908=LINE ( 'NONE', #10163, #13692 ) ;
#7923=AXIS2_PLACEMENT_3D ( 'NONE', #10206, #11214, #10046 ) ;
#7934=AXIS2_PLACEMENT_3D ( 'NONE', #5172, #3829, #10229 ) ;
#7947=EDGE_CURVE ( 'NONE', #11302, #10383, #3325, .T. ) ;
#7950=CARTESIAN_POINT ( 'NONE',  ( 2.500000000000000000, 242.0000000000000284, 40.00000000000000000 ) ) ;
#7965=EDGE_LOOP ( 'NONE', ( #9323, #2918, #4481, #7718, #2110 ) ) ;
#8002=CARTESIAN_POINT ( 'NONE',  ( -0.5000000000000000000, 242.0000000000000284, -47.99999999999999289 ) ) ;
#8019=B_SPLINE_CURVE_WITH_KNOTS ( 'NONE', 3,
 ( #10462, #9221, #6572, #14189 ),
 .UNSPECIFIED., .F., .F.,
 ( 4, 4 ),
 ( 0.009967034006374431848, 0.01711986125270675840 ),
 .UNSPECIFIED. ) ;
#8031=DIRECTION ( 'NONE',  ( 0.000000000000000000, 1.000000000000000000, 0.000000000000000000 ) ) ;
#8035=EDGE_CURVE ( 'NONE', #6499, #16264, #6913, .T. ) ;
#8038=ORIENTED_EDGE ( 'NONE', *, *, #9262, .T. ) ;
#8059=VERTEX_POINT ( 'NONE', #11674 ) ;
#8102=ORIENTED_EDGE ( 'NONE', *, *, #13920, .T. ) ;
#8106=DIRECTION ( 'NONE',  ( -1.000000000000000000, 0.000000000000000000, -0.000000000000000000 ) ) ;
#8122=AXIS2_PLACEMENT_3D ( 'NONE', #6348, #11415, #2673 ) ;
#8125=PRODUCT ( 'Lid Filler Cap _ Measuring Cup', 'Lid Filler Cap _ Measuring Cup', '', ( #6727 ) ) ;
#8138=COLOUR_RGB ( '', 0.09019608, 0.27058824, 0.51372549) ;
#8150=EDGE_CURVE ( 'NONE', #871, #9545, #8480, .T. ) ;
#8165=EDGE_CURVE ( 'NONE', #11431, #2476, #13708, .T. ) ;
#8175=ORIENTED_EDGE ( 'NONE', *, *, #9362, .T. ) ;
#8239=CARTESIAN_POINT ( 'NONE',  ( -2.500000000000000000, 247.0000000000000284, -40.00000000000000000 ) ) ;
#8269=EDGE_CURVE ( 'NONE', #7797, #5335, #1544, .T. ) ;
#8287=ORIENTED_EDGE ( 'NONE', *, *, #1358, .F. ) ;
#8296=CARTESIAN_POINT ( 'NONE',  ( -2.500000000000000000, 247.0000000000000284, 47.99999999999999289 ) ) ;
#8309=EDGE_LOOP ( 'NONE', ( #8513, #10464, #8841, #2626 ) ) ;
#8313=ORIENTED_EDGE ( 'NONE', *, *, #8383, .F. ) ;
#8317=CARTESIAN_POINT ( 'NONE',  ( 43.87482193696061472, 267.0000000000000000, 10.00000000000000178 ) ) ;
#8362=DIRECTION ( 'NONE',  ( 0.000000000000000000, -1.000000000000000000, -0.000000000000000000 ) ) ;
#8383=EDGE_CURVE ( 'NONE', #5335, #6657, #7621, .T. ) ;
#8386=VERTEX_POINT ( 'NONE', #1454 ) ;
#8395=VECTOR ( 'NONE', #958, 1000.000000000000000 ) ;
#8434=EDGE_CURVE ( 'NONE', #9682, #7797, #15671, .T. ) ;
#8451=EDGE_LOOP ( 'NONE', ( #9456, #15363, #14353, #2122 ) ) ;
#8455=EDGE_LOOP ( 'NONE', ( #6017, #10057 ) ) ;
#8480=LINE ( 'NONE', #9819, #6233 ) ;
#8498=DIRECTION ( 'NONE',  ( -0.000000000000000000, -1.000000000000000000, -0.000000000000000000 ) ) ;
#8513=ORIENTED_EDGE ( 'NONE', *, *, #4074, .T. ) ;
#8515=VERTEX_POINT ( 'NONE', #12317 ) ;
#8527=EDGE_LOOP ( 'NONE', ( #8819, #10948, #13140, #6136, #12564, #5, #13580, #8953, #10722, #6280, #10791, #12435, #4799, #10025, #229, #14464, #10812, #13616, #12526, #14842 ) ) ;
#8552=CARTESIAN_POINT ( 'NONE',  ( 5.510910596163089556E-15, 217.0000000000000284, -45.00000000000000000 ) ) ;
#8560=DIRECTION ( 'NONE',  ( 1.000000000000000000, 0.000000000000000000, 0.000000000000000000 ) ) ;
#8617=SURFACE_STYLE_USAGE ( .BOTH. , #6392 ) ;
#8623=ORIENTED_EDGE ( 'NONE', *, *, #5916, .T. ) ;
#8633=DIRECTION ( 'NONE',  ( 0.000000000000000000, -1.000000000000000000, 0.000000000000000000 ) ) ;
#8640=AXIS2_PLACEMENT_3D ( 'NONE', #1865, #3036, #14344 ) ;
#8652=B_SPLINE_CURVE_WITH_KNOTS ( 'NONE', 3,
 ( #15301, #3923, #14053, #6259 ),
 .UNSPECIFIED., .F., .F.,
 ( 4, 4 ),
 ( 0.009967034006374431848, 0.01711986125270675146 ),
 .UNSPECIFIED. ) ;
#8657=AXIS2_PLACEMENT_3D ( 'NONE', #3347, #2251, #12414 ) ;
#8659=ORIENTED_EDGE ( 'NONE', *, *, #1633, .T. ) ;
#8670=VECTOR ( 'NONE', #256, 1000.000000000000000 ) ;
#8683=ORIENTED_EDGE ( 'NONE', *, *, #10581, .F. ) ;
#8684=EDGE_CURVE ( 'NONE', #16436, #2250, #5183, .T. ) ;
#8692=( BOUNDED_CURVE ( )  B_SPLINE_CURVE ( 3, ( #8296, #14680, #5978, #3400 ),
 .UNSPECIFIED., .F., .T. ) 
 B_SPLINE_CURVE_WITH_KNOTS ( ( 4, 4 ),
 ( 3.141592653589793116, 4.712388980384689674 ),
 .UNSPECIFIED. ) 
 CURVE ( )  GEOMETRIC_REPRESENTATION_ITEM ( )  RATIONAL_B_SPLINE_CURVE ( ( 1.000000000000000000, 0.8047378541243649375, 0.8047378541243649375, 1.000000000000000000 ) ) 
 REPRESENTATION_ITEM ( '' )  );
#8720=CARTESIAN_POINT ( 'NONE',  ( -2.500000000000000000, 247.0000000000000284, -47.99999999999999289 ) ) ;
#8769=LINE ( 'NONE', #6452, #3076 ) ;
#8775=EDGE_CURVE ( 'NONE', #15423, #11431, #7041, .T. ) ;
#8781=ORIENTED_EDGE ( 'NONE', *, *, #5987, .T. ) ;
#8796=EDGE_CURVE ( 'NONE', #9638, #13296, #9492, .T. ) ;
#8809=CARTESIAN_POINT ( 'NONE',  ( -0.5000000000000000000, 245.0000000000000284, -49.99999999999999289 ) ) ;
#8810=CARTESIAN_POINT ( 'NONE',  ( 0.000000000000000000, 261.9999999999999432, 0.000000000000000000 ) ) ;
#8819=ORIENTED_EDGE ( 'NONE', *, *, #8165, .F. ) ;
#8820=CARTESIAN_POINT ( 'NONE',  ( -43.87482193696061472, 267.0000000000000000, 10.00000000000000178 ) ) ;
#8841=ORIENTED_EDGE ( 'NONE', *, *, #11380, .F. ) ;
#8847=ADVANCED_FACE ( 'NONE', ( #13544, #9737 ), #12140, .F. ) ;
#8862=VECTOR ( 'NONE', #9744, 1000.000000000000000 ) ;
#8868=DIRECTION ( 'NONE',  ( 0.000000000000000000, -1.000000000000000000, 0.000000000000000000 ) ) ;
#8873=AXIS2_PLACEMENT_3D ( 'NONE', #1815, #4324, #6907 ) ;
#8876=EDGE_CURVE ( 'NONE', #11431, #15423, #115, .T. ) ;
#8908=ORIENTED_EDGE ( 'NONE', *, *, #1924, .T. ) ;
#8922=VECTOR ( 'NONE', #6601, 1000.000000000000000 ) ;
#8932=EDGE_LOOP ( 'NONE', ( #1805, #13923, #8683, #4943 ) ) ;
#8943=DIRECTION ( 'NONE',  ( -0.000000000000000000, -1.000000000000000000, -0.000000000000000000 ) ) ;
#8953=ORIENTED_EDGE ( 'NONE', *, *, #9362, .F. ) ;
#8955=PLANE ( 'NONE',  #935 ) ;
#8963=PRESENTATION_STYLE_ASSIGNMENT (( #8617 ) ) ;
#8964=CARTESIAN_POINT ( 'NONE',  ( 2.500000000000000000, 247.0000000000000284, 47.99999999999999289 ) ) ;
#8967=VERTEX_POINT ( 'NONE', #2480 ) ;
#8987=( NAMED_UNIT ( * ) PLANE_ANGLE_UNIT ( ) SI_UNIT ( $, .RADIAN. ) );
#8993=CARTESIAN_POINT ( 'NONE',  ( -45.00000000000000000, 262.0000000000000000, -10.00000000000000178 ) ) ;
#8995=CARTESIAN_POINT ( 'NONE',  ( 0.000000000000000000, 242.0000000000000284, 0.000000000000000000 ) ) ;
#8998=CARTESIAN_POINT ( 'NONE',  ( 0.000000000000000000, 217.0000000000000284, 45.00000000000000000 ) ) ;
#9026=DIRECTION ( 'NONE',  ( 0.000000000000000000, 0.000000000000000000, 1.000000000000000000 ) ) ;
#9033=VERTEX_POINT ( 'NONE', #8720 ) ;
#9045=CARTESIAN_POINT ( 'NONE',  ( 2.500000000000000000, 247.0000000000000284, -47.99999999999999289 ) ) ;
#9052=FACE_OUTER_BOUND ( 'NONE', #1704, .T. ) ;
#9054=ORIENTED_EDGE ( 'NONE', *, *, #7778, .T. ) ;
#9070=CARTESIAN_POINT ( 'NONE',  ( -2.500000000000000000, 247.0000000000000284, -47.99999999999999289 ) ) ;
#9129=CYLINDRICAL_SURFACE ( 'NONE', #6825, 2.000000000000001776 ) ;
#9133=EDGE_CURVE ( 'NONE', #10385, #11502, #6521, .T. ) ;
#9135=DIRECTION ( 'NONE',  ( -0.000000000000000000, 1.000000000000000000, -0.000000000000000000 ) ) ;
#9158=LINE ( 'NONE', #8998, #8922 ) ;
#9188=AXIS2_PLACEMENT_3D ( 'NONE', #5834, #12398, #3581 ) ;
#9208=( BOUNDED_CURVE ( )  B_SPLINE_CURVE ( 3, ( #2264, #7274, #14645, #9849 ),
 .UNSPECIFIED., .F., .T. ) 
 B_SPLINE_CURVE_WITH_KNOTS ( ( 4, 4 ),
 ( 4.712388980384689674, 6.283185307179586232 ),
 .UNSPECIFIED. ) 
 CURVE ( )  GEOMETRIC_REPRESENTATION_ITEM ( )  RATIONAL_B_SPLINE_CURVE ( ( 1.000000000000000000, 0.8047378541243649375, 0.8047378541243649375, 1.000000000000000000 ) ) 
 REPRESENTATION_ITEM ( '' )  );
#9221=CARTESIAN_POINT ( 'NONE',  ( -45.58196769024076644, 258.6644603543468861, -10.00000000000000178 ) ) ;
#9232=DIRECTION ( 'NONE',  ( 0.000000000000000000, 0.000000000000000000, -1.000000000000000000 ) ) ;
#9262=EDGE_CURVE ( 'NONE', #8059, #7640, #13118, .T. ) ;
#9265=FACE_OUTER_BOUND ( 'NONE', #8451, .T. ) ;
#9288=CYLINDRICAL_SURFACE ( 'NONE', #8640, 45.00000000000000000 ) ;
#9292=CARTESIAN_POINT ( 'NONE',  ( 0.000000000000000000, 247.0000000000000284, 0.000000000000000000 ) ) ;
#9315=CARTESIAN_POINT ( 'NONE',  ( 0.000000000000000000, 261.9999999999999432, 49.99999999999999289 ) ) ;
#9322=ORIENTED_EDGE ( 'NONE', *, *, #11292, .F. ) ;
#9323=ORIENTED_EDGE ( 'NONE', *, *, #9772, .T. ) ;
#9357=EDGE_CURVE ( 'NONE', #2833, #8386, #6660, .T. ) ;
#9361=ORIENTED_EDGE ( 'NONE', *, *, #1633, .F. ) ;
#9362=EDGE_CURVE ( 'NONE', #9544, #5908, #16074, .T. ) ;
#9376=CIRCLE ( 'NONE', #4339, 45.00000000000000000 ) ;
#9383=DIRECTION ( 'NONE',  ( 0.000000000000000000, -1.000000000000000000, 0.000000000000000000 ) ) ;
#9399=ORIENTED_EDGE ( 'NONE', *, *, #8684, .T. ) ;
#9400=ORIENTED_EDGE ( 'NONE', *, *, #7058, .F. ) ;
#9415=VECTOR ( 'NONE', #5702, 1000.000000000000000 ) ;
#9435=AXIS2_PLACEMENT_3D ( 'NONE', #9292, #8031, #5564 ) ;
#9454=VECTOR ( 'NONE', #14849, 1000.000000000000000 ) ;
#9455=CIRCLE ( 'NONE', #11581, 45.00000000000000000 ) ;
#9456=ORIENTED_EDGE ( 'NONE', *, *, #8434, .T. ) ;
#9461=ORIENTED_EDGE ( 'NONE', *, *, #13222, .T. ) ;
#9467=AXIS2_PLACEMENT_3D ( 'NONE', #260, #15562, #6861 ) ;
#9481=DIRECTION ( 'NONE',  ( 0.000000000000000000, 0.000000000000000000, -1.000000000000000000 ) ) ;
#9492=LINE ( 'NONE', #1825, #7304 ) ;
#9493=ORIENTED_EDGE ( 'NONE', *, *, #1358, .T. ) ;
#9511=CARTESIAN_POINT ( 'NONE',  ( -43.87482193696060762, 257.0000000000001137, 10.00000000000000178 ) ) ;
#9544=VERTEX_POINT ( 'NONE', #628 ) ;
#9545=VERTEX_POINT ( 'NONE', #5725 ) ;
#9551=CIRCLE ( 'NONE', #4518, 49.99999999999999289 ) ;
#9557=CARTESIAN_POINT ( 'NONE',  ( 2.500000000000000000, 242.0000000000000284, -47.99999999999999289 ) ) ;
#9566=EDGE_LOOP ( 'NONE', ( #12197, #13679, #9812 ) ) ;
#9590=CARTESIAN_POINT ( 'NONE',  ( 0.000000000000000000, 247.0000000000000284, 45.00000000000000000 ) ) ;
#9593=CARTESIAN_POINT ( 'NONE',  ( 0.000000000000000000, 245.0000000000000284, 47.99999999999999289 ) ) ;
#9605=EDGE_LOOP ( 'NONE', ( #3781, #10994 ) ) ;
#9610=ADVANCED_FACE ( 'NONE', ( #43 ), #8955, .F. ) ;
#9629=DIRECTION ( 'NONE',  ( 0.000000000000000000, 1.000000000000000000, 0.000000000000000000 ) ) ;
#9635=ADVANCED_FACE ( 'NONE', ( #2380 ), #16266, .T. ) ;
#9638=VERTEX_POINT ( 'NONE', #10044 ) ;
#9663=ORIENTED_EDGE ( 'NONE', *, *, #8150, .T. ) ;
#9668=DIRECTION ( 'NONE',  ( -0.000000000000000000, -1.000000000000000000, -0.000000000000000000 ) ) ;
#9682=VERTEX_POINT ( 'NONE', #10203 ) ;
#9737=FACE_BOUND ( 'NONE', #7154, .T. ) ;
#9738=CIRCLE ( 'NONE', #1764, 45.00000000000000000 ) ;
#9744=DIRECTION ( 'NONE',  ( -0.000000000000000000, -1.000000000000000000, -0.000000000000000000 ) ) ;
#9764=DIRECTION ( 'NONE',  ( 0.000000000000000000, 0.000000000000000000, -1.000000000000000000 ) ) ;
#9772=EDGE_CURVE ( 'NONE', #9937, #16264, #6718, .T. ) ;
#9794=ORIENTED_EDGE ( 'NONE', *, *, #11634, .T. ) ;
#9812=ORIENTED_EDGE ( 'NONE', *, *, #8684, .F. ) ;
#9813=ORIENTED_EDGE ( 'NONE', *, *, #10873, .F. ) ;
#9819=CARTESIAN_POINT ( 'NONE',  ( 2.500000000000000000, 242.0000000000000284, -40.00000000000000000 ) ) ;
#9826=ADVANCED_FACE ( 'NONE', ( #12945 ), #13187, .F. ) ;
#9849=CARTESIAN_POINT ( 'NONE',  ( -2.500000000000000000, 242.0000000000000284, -47.99999999999999289 ) ) ;
#9901=DIRECTION ( 'NONE',  ( -0.000000000000000000, 1.000000000000000000, -0.000000000000000000 ) ) ;
#9919=CARTESIAN_POINT ( 'NONE',  ( 0.000000000000000000, 217.0000000000000284, 40.00000000000000000 ) ) ;
#9922=DIRECTION ( 'NONE',  ( 0.000000000000000000, 0.000000000000000000, -1.000000000000000000 ) ) ;
#9937=VERTEX_POINT ( 'NONE', #15599 ) ;
#9962=LINE ( 'NONE', #10959, #15578 ) ;
#9966=ORIENTED_EDGE ( 'NONE', *, *, #14122, .F. ) ;
#9967=AXIS2_PLACEMENT_3D ( 'NONE', #2902, #13042, #802 ) ;
#9970=ORIENTED_EDGE ( 'NONE', *, *, #11292, .T. ) ;
#9982=CARTESIAN_POINT ( 'NONE',  ( 1.671572875253809487, 246.1715728752537871, 50.00000000000000000 ) ) ;
#9998=AXIS2_PLACEMENT_3D ( 'NONE', #5357, #12985, #15467 ) ;
#10002=DIRECTION ( 'NONE',  ( 0.000000000000000000, 0.000000000000000000, -1.000000000000000000 ) ) ;
#10012=AXIS2_PLACEMENT_3D ( 'NONE', #6415, #12647, #4774 ) ;
#10025=ORIENTED_EDGE ( 'NONE', *, *, #12949, .F. ) ;
#10029=LINE ( 'NONE', #105, #13648 ) ;
#10035=ADVANCED_FACE ( 'NONE', ( #6181 ), #16232, .F. ) ;
#10044=CARTESIAN_POINT ( 'NONE',  ( -2.500000000000000000, 242.0000000000000284, -44.93050188902856945 ) ) ;
#10046=DIRECTION ( 'NONE',  ( 0.000000000000000000, 0.000000000000000000, 1.000000000000000000 ) ) ;
#10056=EDGE_LOOP ( 'NONE', ( #11914, #9399, #11521, #9970, #9493 ) ) ;
#10057=ORIENTED_EDGE ( 'NONE', *, *, #15858, .F. ) ;
#10058=ORIENTED_EDGE ( 'NONE', *, *, #11093, .F. ) ;
#10071=DIRECTION ( 'NONE',  ( 0.000000000000000000, 1.000000000000000000, 0.000000000000000000 ) ) ;
#10104=ORIENTED_EDGE ( 'NONE', *, *, #4039, .F. ) ;
#10112=CARTESIAN_POINT ( 'NONE',  ( 2.500000000000000000, 244.0000000000000284, 49.99999999999999289 ) ) ;
#10148=DIRECTION ( 'NONE',  ( 0.000000000000000000, 1.000000000000000000, 0.000000000000000000 ) ) ;
#10163=CARTESIAN_POINT ( 'NONE',  ( 0.000000000000000000, 217.0000000000000284, 45.00000000000000000 ) ) ;
#10192=LINE ( 'NONE', #12597, #697 ) ;
#10203=CARTESIAN_POINT ( 'NONE',  ( 0.5000000000000000000, 244.0000000000000284, -49.99999999999999289 ) ) ;
#10206=CARTESIAN_POINT ( 'NONE',  ( 0.000000000000000000, 257.0000000000001137, 0.000000000000000000 ) ) ;
#10229=DIRECTION ( 'NONE',  ( 0.000000000000000000, 0.000000000000000000, 1.000000000000000000 ) ) ;
#10252=B_SPLINE_CURVE_WITH_KNOTS ( 'NONE', 3,
 ( #6940, #4358, #11992, #9511 ),
 .UNSPECIFIED., .F., .F.,
 ( 4, 4 ),
 ( 0.01002676606614814371, 0.01717959331248046853 ),
 .UNSPECIFIED. ) ;
#10262=UNCERTAINTY_MEASURE_WITH_UNIT (LENGTH_MEASURE( 1.000000000000000082E-05 ), #1216, 'distance_accuracy_value', 'NONE');
#10283=CIRCLE ( 'NONE', #14494, 45.00000000000000000 ) ;
#10284=ADVANCED_FACE ( 'NONE', ( #15305 ), #7582, .F. ) ;
#10344=EDGE_LOOP ( 'NONE', ( #5295, #4256, #6696, #16185, #14257 ) ) ;
#10353=LINE ( 'NONE', #10112, #4448 ) ;
#10383=VERTEX_POINT ( 'NONE', #15712 ) ;
#10385=VERTEX_POINT ( 'NONE', #573 ) ;
#10401=FILL_AREA_STYLE_COLOUR ( '', #8138 ) ;
#10410=ORIENTED_EDGE ( 'NONE', *, *, #15858, .T. ) ;
#10459=ORIENTED_EDGE ( 'NONE', *, *, #6967, .F. ) ;
#10462=CARTESIAN_POINT ( 'NONE',  ( -43.87482193696061472, 257.0000000000001137, -10.00000000000000178 ) ) ;
#10464=ORIENTED_EDGE ( 'NONE', *, *, #2650, .T. ) ;
#10467=CONICAL_SURFACE ( 'NONE', #6223, 49.99999999999999289, 0.7853981633974642662 ) ;
#10516=CARTESIAN_POINT ( 'NONE',  ( 2.500000000000000000, 242.0000000000000284, 47.99999999999999289 ) ) ;
#10518=ADVANCED_FACE ( 'NONE', ( #4583 ), #15008, .T. ) ;
#10543=EDGE_CURVE ( 'NONE', #8515, #7197, #16213, .T. ) ;
#10545=PLANE ( 'NONE',  #9435 ) ;
#10558=AXIS2_PLACEMENT_3D ( 'NONE', #1911, #2161, #3510 ) ;
#10562=CARTESIAN_POINT ( 'NONE',  ( -45.00000000000000000, 262.0000000000000000, 10.00000000000000178 ) ) ;
#10581=EDGE_CURVE ( 'NONE', #7494, #2831, #11463, .T. ) ;
#10594=DIRECTION ( 'NONE',  ( 0.000000000000000000, 0.000000000000000000, -1.000000000000000000 ) ) ;
#10603=DIRECTION ( 'NONE',  ( -0.000000000000000000, 1.000000000000000000, -0.000000000000000000 ) ) ;
#10618=EDGE_CURVE ( 'NONE', #6571, #8515, #7083, .T. ) ;
#10620=CARTESIAN_POINT ( 'NONE',  ( 0.000000000000000000, 247.0000000000000284, 0.000000000000000000 ) ) ;
#10630=DIRECTION ( 'NONE',  ( 0.000000000000000000, 0.000000000000000000, -1.000000000000000000 ) ) ;
#10635=ORIENTED_EDGE ( 'NONE', *, *, #9772, .F. ) ;
#10650=ORIENTED_EDGE ( 'NONE', *, *, #7766, .T. ) ;
#10657=ORIENTED_EDGE ( 'NONE', *, *, #15660, .F. ) ;
#10662=ADVANCED_FACE ( 'NONE', ( #13549 ), #10899, .F. ) ;
#10668=CARTESIAN_POINT ( 'NONE',  ( -2.499999999999999556, 247.0000000000000568, -49.17157287525380127 ) ) ;
#10676=DIRECTION ( 'NONE',  ( -1.000000000000000000, 0.000000000000000000, -0.000000000000000000 ) ) ;
#10703=VECTOR ( 'NONE', #14885, 1000.000000000000000 ) ;
#10722=ORIENTED_EDGE ( 'NONE', *, *, #6886, .F. ) ;
#10724=ORIENTED_EDGE ( 'NONE', *, *, #14051, .T. ) ;
#10781=CARTESIAN_POINT ( 'NONE',  ( 43.87482193696061472, 262.0000000000000000, 10.00000000000000178 ) ) ;
#10791=ORIENTED_EDGE ( 'NONE', *, *, #13129, .T. ) ;
#10795=VERTEX_POINT ( 'NONE', #2574 ) ;
#10801=FACE_BOUND ( 'NONE', #2295, .T. ) ;
#10804=VECTOR ( 'NONE', #6979, 1000.000000000000000 ) ;
#10812=ORIENTED_EDGE ( 'NONE', *, *, #5987, .F. ) ;
#10854=ORIENTED_EDGE ( 'NONE', *, *, #407, .F. ) ;
#10870=ORIENTED_EDGE ( 'NONE', *, *, #11634, .F. ) ;
#10873=EDGE_CURVE ( 'NONE', #9033, #13296, #149, .T. ) ;
#10890=EDGE_LOOP ( 'NONE', ( #13901, #7722, #5721, #13883 ) ) ;
#10899=PLANE ( 'NONE',  #3896 ) ;
#10900=DIRECTION ( 'NONE',  ( -0.000000000000000000, -0.000000000000000000, -1.000000000000000000 ) ) ;
#10948=ORIENTED_EDGE ( 'NONE', *, *, #8775, .F. ) ;
#10959=CARTESIAN_POINT ( 'NONE',  ( 0.000000000000000000, 217.0000000000000284, 45.00000000000000000 ) ) ;
#10994=ORIENTED_EDGE ( 'NONE', *, *, #8876, .T. ) ;
#11036=EDGE_CURVE ( 'NONE', #1977, #5468, #9738, .T. ) ;
#11055=ORIENTED_EDGE ( 'NONE', *, *, #2965, .T. ) ;
#11070=DIRECTION ( 'NONE',  ( 1.000000000000000000, 0.000000000000000000, 0.000000000000000000 ) ) ;
#11073=DIRECTION ( 'NONE',  ( 0.000000000000000000, 0.000000000000000000, 1.000000000000000000 ) ) ;
#11093=EDGE_CURVE ( 'NONE', #11111, #11502, #6618, .T. ) ;
#11111=VERTEX_POINT ( 'NONE', #516 ) ;
#11120=EDGE_CURVE ( 'NONE', #4312, #9544, #10252, .T. ) ;
#11125=ADVANCED_FACE ( 'NONE', ( #5449 ), #3183, .T. ) ;
#11138=CARTESIAN_POINT ( 'NONE',  ( -2.500000000000000000, 242.0000000000000284, 47.99999999999999289 ) ) ;
#11147=VERTEX_POINT ( 'NONE', #9590 ) ;
#11167=ADVANCED_FACE ( 'NONE', ( #14470 ), #15655, .T. ) ;
#11202=ADVANCED_FACE ( 'NONE', ( #9265 ), #14321, .T. ) ;
#11209=EDGE_CURVE ( 'NONE', #7494, #16264, #5540, .T. ) ;
#11214=DIRECTION ( 'NONE',  ( 0.000000000000000000, 1.000000000000000000, 0.000000000000000000 ) ) ;
#11263=VECTOR ( 'NONE', #15197, 1000.000000000000000 ) ;
#11292=EDGE_CURVE ( 'NONE', #8059, #11111, #3626, .T. ) ;
#11302=VERTEX_POINT ( 'NONE', #9919 ) ;
#11315=VECTOR ( 'NONE', #9901, 1000.000000000000000 ) ;
#11344=FACE_OUTER_BOUND ( 'NONE', #3687, .T. ) ;
#11352=VECTOR ( 'NONE', #15127, 1000.000000000000000 ) ;
#11374=CARTESIAN_POINT ( 'NONE',  ( 0.000000000000000000, 217.0000000000000284, 0.000000000000000000 ) ) ;
#11376=EDGE_CURVE ( 'NONE', #3456, #1328, #15824, .T. ) ;
#11380=EDGE_CURVE ( 'NONE', #10383, #13787, #1491, .T. ) ;
#11381=CARTESIAN_POINT ( 'NONE',  ( 0.000000000000000000, 262.0000000000000000, 45.00000000000000000 ) ) ;
#11404=VERTEX_POINT ( 'NONE', #16059 ) ;
#11415=DIRECTION ( 'NONE',  ( -0.000000000000000000, 1.000000000000000000, -0.000000000000000000 ) ) ;
#11422=CARTESIAN_POINT ( 'NONE',  ( -2.500000000000000000, 247.0000000000000284, -47.99999999999999289 ) ) ;
#11431=VERTEX_POINT ( 'NONE', #3839 ) ;
#11446=ORIENTED_EDGE ( 'NONE', *, *, #10618, .F. ) ;
#11463=( BOUNDED_CURVE ( )  B_SPLINE_CURVE ( 3, ( #3420, #15041, #9982, #6089 ),
 .UNSPECIFIED., .F., .F. ) 
 B_SPLINE_CURVE_WITH_KNOTS ( ( 4, 4 ),
 ( 0.000000000000000000, 1.570796326794896558 ),
 .UNSPECIFIED. ) 
 CURVE ( )  GEOMETRIC_REPRESENTATION_ITEM ( )  RATIONAL_B_SPLINE_CURVE ( ( 1.000000000000000000, 0.8047378541243649375, 0.8047378541243649375, 1.000000000000000000 ) ) 
 REPRESENTATION_ITEM ( '' )  );
#11496=ADVANCED_FACE ( 'NONE', ( #13884 ), #7821, .F. ) ;
#11502=VERTEX_POINT ( 'NONE', #14130 ) ;
#11514=LINE ( 'NONE', #15415, #5773 ) ;
#11521=ORIENTED_EDGE ( 'NONE', *, *, #12949, .T. ) ;
#11549=CARTESIAN_POINT ( 'NONE',  ( -2.500000000000000000, 242.0000000000000284, 47.99999999999999289 ) ) ;
#11554=FILL_AREA_STYLE ('',( #10401 ) ) ;
#11571=CIRCLE ( 'NONE', #140, 45.00000000000000000 ) ;
#11581=AXIS2_PLACEMENT_3D ( 'NONE', #10620, #7426, #1167 ) ;
#11632=ORIENTED_EDGE ( 'NONE', *, *, #10873, .T. ) ;
#11634=EDGE_CURVE ( 'NONE', #14317, #3456, #8652, .T. ) ;
#11635=DIRECTION ( 'NONE',  ( 0.000000000000000000, 0.000000000000000000, 1.000000000000000000 ) ) ;
#11659=EDGE_CURVE ( 'NONE', #6571, #3157, #10283, .T. ) ;
#11674=CARTESIAN_POINT ( 'NONE',  ( 5.510910596163089556E-15, 262.0000000000000000, -45.00000000000000000 ) ) ;
#11685=DIRECTION ( 'NONE',  ( 0.000000000000000000, 1.000000000000000000, 0.000000000000000000 ) ) ;
#11710=DIRECTION ( 'NONE',  ( 0.000000000000000000, -1.000000000000000000, 0.000000000000000000 ) ) ;
#11720=FACE_OUTER_BOUND ( 'NONE', #15077, .T. ) ;
#11725=ORIENTED_EDGE ( 'NONE', *, *, #15831, .F. ) ;
#11731=DIRECTION ( 'NONE',  ( 0.000000000000000000, -1.000000000000000000, 0.000000000000000000 ) ) ;
#11825=VECTOR ( 'NONE', #9135, 1000.000000000000000 ) ;
#11837=AXIS2_PLACEMENT_3D ( 'NONE', #12571, #7500, #9922 ) ;
#11855=DIRECTION ( 'NONE',  ( 0.000000000000000000, 0.000000000000000000, 1.000000000000000000 ) ) ;
#11880=CARTESIAN_POINT ( 'NONE',  ( 0.000000000000000000, 217.0000000000000284, 0.000000000000000000 ) ) ;
#11881=LINE ( 'NONE', #478, #10804 ) ;
#11884=CARTESIAN_POINT ( 'NONE',  ( 2.500000000000000000, 244.0000000000000284, -47.99999999999999289 ) ) ;
#11892=ORIENTED_EDGE ( 'NONE', *, *, #13214, .F. ) ;
#11911=ADVANCED_FACE ( 'NONE', ( #3322 ), #3576, .T. ) ;
#11914=ORIENTED_EDGE ( 'NONE', *, *, #2965, .F. ) ;
#11941=AXIS2_PLACEMENT_3D ( 'NONE', #5089, #6487, #12476 ) ;
#11992=CARTESIAN_POINT ( 'NONE',  ( -45.58196769024076644, 258.6644603543468861, 10.00000000000000178 ) ) ;
#12026=EDGE_LOOP ( 'NONE', ( #6985, #11632, #16435, #12340 ) ) ;
#12036=CARTESIAN_POINT ( 'NONE',  ( 1.671572875253809487, 242.8284271247462129, -49.99999999999999289 ) ) ;
#12044=ORIENTED_EDGE ( 'NONE', *, *, #12934, .T. ) ;
#12051=ORIENTED_EDGE ( 'NONE', *, *, #15914, .T. ) ;
#12067=UNCERTAINTY_MEASURE_WITH_UNIT (LENGTH_MEASURE( 1.000000000000000082E-05 ), #2386, 'distance_accuracy_value', 'NONE');
#12140=PLANE ( 'NONE',  #16326 ) ;
#12195=ORIENTED_EDGE ( 'NONE', *, *, #11120, .F. ) ;
#12197=ORIENTED_EDGE ( 'NONE', *, *, #99, .F. ) ;
#12208=FACE_OUTER_BOUND ( 'NONE', #7965, .T. ) ;
#12213=DIRECTION ( 'NONE',  ( -0.000000000000000000, -1.000000000000000000, -0.000000000000000000 ) ) ;
#12253=ADVANCED_FACE ( 'NONE', ( #4063 ), #13279, .T. ) ;
#12290=EDGE_LOOP ( 'NONE', ( #7715, #13940, #7163, #14921 ) ) ;
#12291=ADVANCED_FACE ( 'NONE', ( #5643 ), #15768, .T. ) ;
#12317=CARTESIAN_POINT ( 'NONE',  ( -2.500000000000000000, 247.0000000000000284, 44.93050188902856945 ) ) ;
#12340=ORIENTED_EDGE ( 'NONE', *, *, #15226, .T. ) ;
#12369=PLANE ( 'NONE',  #4437 ) ;
#12373=CIRCLE ( 'NONE', #7075, 45.00000000000000000 ) ;
#12378=APPLICATION_CONTEXT ( 'automotive_design' ) ;
#12398=DIRECTION ( 'NONE',  ( 0.000000000000000000, 1.000000000000000000, 0.000000000000000000 ) ) ;
#12414=DIRECTION ( 'NONE',  ( 0.000000000000000000, 0.000000000000000000, -1.000000000000000000 ) ) ;
#12435=ORIENTED_EDGE ( 'NONE', *, *, #13167, .T. ) ;
#12465=ORIENTED_EDGE ( 'NONE', *, *, #716, .F. ) ;
#12476=DIRECTION ( 'NONE',  ( 1.000000000000000000, 0.000000000000000000, 0.000000000000000000 ) ) ;
#12478=CARTESIAN_POINT ( 'NONE',  ( 43.87482193696061472, 267.0000000000000000, 10.00000000000000178 ) ) ;
#12526=ORIENTED_EDGE ( 'NONE', *, *, #15226, .F. ) ;
#12535=CARTESIAN_POINT ( 'NONE',  ( 2.500000000000000000, 247.0000000000000284, -44.93050188902856945 ) ) ;
#12554=CIRCLE ( 'NONE', #53, 49.99999999999999289 ) ;
#12564=ORIENTED_EDGE ( 'NONE', *, *, #10618, .T. ) ;
#12571=CARTESIAN_POINT ( 'NONE',  ( -45.00000000000000000, 262.0000000000000000, 0.000000000000000000 ) ) ;
#12578=CARTESIAN_POINT ( 'NONE',  ( 2.500000000000000000, 217.0000000000000284, 44.93050188902856945 ) ) ;
#12592=CARTESIAN_POINT ( 'NONE',  ( -0.5000000000000000000, 244.0000000000000284, -49.99999999999999289 ) ) ;
#12597=CARTESIAN_POINT ( 'NONE',  ( -43.87482193696061472, 267.0000000000000000, -10.00000000000000178 ) ) ;
#12606=EDGE_LOOP ( 'NONE', ( #13113, #4392, #13904, #9054, #4802, #8781, #4393, #10058, #9322, #8038, #10410, #13765, #4496, #3345, #10854, #7556, #12044, #15686, #9966, #11892 ) ) ;
#12612=CYLINDRICAL_SURFACE ( 'NONE', #7593, 45.00000000000000000 ) ;
#12619=DIRECTION ( 'NONE',  ( -0.000000000000000000, -0.000000000000000000, -1.000000000000000000 ) ) ;
#12637=LINE ( 'NONE', #3828, #11263 ) ;
#12647=DIRECTION ( 'NONE',  ( 0.000000000000000000, 1.000000000000000000, 0.000000000000000000 ) ) ;
#12654=CIRCLE ( 'NONE', #9998, 45.00000000000000000 ) ;
#12655=AXIS2_PLACEMENT_3D ( 'NONE', #2940, #7015, #1686 ) ;
#12765=FACE_OUTER_BOUND ( 'NONE', #14616, .T. ) ;
#12833=ORIENTED_EDGE ( 'NONE', *, *, #8150, .F. ) ;
#12851=DIRECTION ( 'NONE',  ( 1.000000000000000000, -0.000000000000000000, -0.000000000000000000 ) ) ;
#12870=CARTESIAN_POINT ( 'NONE',  ( 0.000000000000000000, 245.0000000000000284, -47.99999999999999289 ) ) ;
#12881=DIRECTION ( 'NONE',  ( -0.000000000000000000, 1.000000000000000000, -0.000000000000000000 ) ) ;
#12888=( LENGTH_UNIT ( ) NAMED_UNIT ( * ) SI_UNIT ( .MILLI., .METRE. ) );
#12915=AXIS2_PLACEMENT_3D ( 'NONE', #13380, #333, #14302 ) ;
#12934=EDGE_CURVE ( 'NONE', #11147, #12980, #9455, .T. ) ;
#12943=ORIENTED_EDGE ( 'NONE', *, *, #11376, .T. ) ;
#12945=FACE_OUTER_BOUND ( 'NONE', #9566, .T. ) ;
#12949=EDGE_CURVE ( 'NONE', #2250, #8059, #12373, .T. ) ;
#12970=CIRCLE ( 'NONE', #7923, 45.00000000000000000 ) ;
#12980=VERTEX_POINT ( 'NONE', #7182 ) ;
#12985=DIRECTION ( 'NONE',  ( 0.000000000000000000, -1.000000000000000000, 0.000000000000000000 ) ) ;
#12987=CARTESIAN_POINT ( 'NONE',  ( 0.000000000000000000, 242.0000000000000284, 0.000000000000000000 ) ) ;
#13020=ORIENTED_EDGE ( 'NONE', *, *, #11376, .F. ) ;
#13042=DIRECTION ( 'NONE',  ( 0.000000000000000000, 1.000000000000000000, 0.000000000000000000 ) ) ;
#13076=DIRECTION ( 'NONE',  ( 0.000000000000000000, -1.000000000000000000, 0.000000000000000000 ) ) ;
#13081=DIRECTION ( 'NONE',  ( -0.000000000000000000, 0.000000000000000000, -1.000000000000000000 ) ) ;
#13113=ORIENTED_EDGE ( 'NONE', *, *, #8876, .F. ) ;
#13118=LINE ( 'NONE', #13280, #11825 ) ;
#13123=LINE ( 'NONE', #5413, #14298 ) ;
#13129=EDGE_CURVE ( 'NONE', #1977, #14690, #9158, .T. ) ;
#13137=CARTESIAN_POINT ( 'NONE',  ( 0.000000000000000000, 217.0000000000000284, 0.000000000000000000 ) ) ;
#13140=ORIENTED_EDGE ( 'NONE', *, *, #13214, .T. ) ;
#13163=CARTESIAN_POINT ( 'NONE',  ( 1.671572875253809487, 242.8284271247462129, 49.99999999999999289 ) ) ;
#13167=EDGE_CURVE ( 'NONE', #14690, #7640, #12654, .T. ) ;
#13183=VECTOR ( 'NONE', #6099, 1000.000000000000000 ) ;
#13187=PLANE ( 'NONE',  #6523 ) ;
#13205=FACE_OUTER_BOUND ( 'NONE', #9605, .T. ) ;
#13214=EDGE_CURVE ( 'NONE', #15423, #3157, #7908, .T. ) ;
#13222=EDGE_CURVE ( 'NONE', #13787, #10383, #5498, .T. ) ;
#13226=ORIENTED_EDGE ( 'NONE', *, *, #6218, .T. ) ;
#13227=VECTOR ( 'NONE', #12619, 1000.000000000000000 ) ;
#13261=ORIENTED_EDGE ( 'NONE', *, *, #11209, .F. ) ;
#13279=PLANE ( 'NONE',  #5529 ) ;
#13280=CARTESIAN_POINT ( 'NONE',  ( 5.510910596163089556E-15, 217.0000000000000284, -45.00000000000000000 ) ) ;
#13296=VERTEX_POINT ( 'NONE', #5753 ) ;
#13380=CARTESIAN_POINT ( 'NONE',  ( 0.000000000000000000, 247.0000000000000284, 0.000000000000000000 ) ) ;
#13422=EDGE_CURVE ( 'NONE', #8515, #11147, #3625, .T. ) ;
#13426=STYLED_ITEM ( 'NONE', ( #8963 ), #1465 ) ;
#13447=STYLED_ITEM ( 'NONE', ( #161 ), #14144 ) ;
#13453=CARTESIAN_POINT ( 'NONE',  ( 0.5000000000000000000, 244.0000000000000284, -49.99999999999999289 ) ) ;
#13544=FACE_OUTER_BOUND ( 'NONE', #8455, .T. ) ;
#13549=FACE_OUTER_BOUND ( 'NONE', #5886, .T. ) ;
#13580=ORIENTED_EDGE ( 'NONE', *, *, #13811, .T. ) ;
#13616=ORIENTED_EDGE ( 'NONE', *, *, #6218, .F. ) ;
#13620=DIRECTION ( 'NONE',  ( 0.000000000000000000, 0.000000000000000000, 1.000000000000000000 ) ) ;
#13648=VECTOR ( 'NONE', #3947, 1000.000000000000000 ) ;
#13679=ORIENTED_EDGE ( 'NONE', *, *, #5927, .F. ) ;
#13684=( BOUNDED_CURVE ( )  B_SPLINE_CURVE ( 3, ( #9045, #14100, #7875, #1555 ),
 .UNSPECIFIED., .F., .F. ) 
 B_SPLINE_CURVE_WITH_KNOTS ( ( 4, 4 ),
 ( 0.000000000000000000, 1.570796326794896780 ),
 .UNSPECIFIED. ) 
 CURVE ( )  GEOMETRIC_REPRESENTATION_ITEM ( )  RATIONAL_B_SPLINE_CURVE ( ( 1.000000000000000000, 0.8047378541243649375, 0.8047378541243649375, 1.000000000000000000 ) ) 
 REPRESENTATION_ITEM ( '' )  );
#13690=( NAMED_UNIT ( * ) PLANE_ANGLE_UNIT ( ) SI_UNIT ( $, .RADIAN. ) );
#13692=VECTOR ( 'NONE', #6683, 1000.000000000000000 ) ;
#13708=LINE ( 'NONE', #8552, #6785 ) ;
#13715=LINE ( 'NONE', #11549, #1700 ) ;
#13728=EDGE_CURVE ( 'NONE', #6657, #9682, #11881, .T. ) ;
#13747=ORIENTED_EDGE ( 'NONE', *, *, #10543, .F. ) ;
#13765=ORIENTED_EDGE ( 'NONE', *, *, #13129, .F. ) ;
#13768=DIRECTION ( 'NONE',  ( 0.000000000000000000, 1.000000000000000000, 0.000000000000000000 ) ) ;
#13776=LINE ( 'NONE', #15106, #13227 ) ;
#13787=VERTEX_POINT ( 'NONE', #15620 ) ;
#13802=LINE ( 'NONE', #1245, #13183 ) ;
#13811=EDGE_CURVE ( 'NONE', #11147, #5908, #9962, .T. ) ;
#13846=DIRECTION ( 'NONE',  ( -1.000000000000000000, 0.000000000000000000, -0.000000000000000000 ) ) ;
#13850=ADVANCED_FACE ( 'NONE', ( #12208 ), #12369, .F. ) ;
#13883=ORIENTED_EDGE ( 'NONE', *, *, #9357, .T. ) ;
#13884=FACE_OUTER_BOUND ( 'NONE', #4965, .T. ) ;
#13901=ORIENTED_EDGE ( 'NONE', *, *, #5959, .T. ) ;
#13904=ORIENTED_EDGE ( 'NONE', *, *, #7058, .T. ) ;
#13920=EDGE_CURVE ( 'NONE', #8386, #14589, #1058, .T. ) ;
#13923=ORIENTED_EDGE ( 'NONE', *, *, #2754, .F. ) ;
#13936=CARTESIAN_POINT ( 'NONE',  ( -2.500000000000000000, 242.0000000000000284, 47.99999999999999289 ) ) ;
#13940=ORIENTED_EDGE ( 'NONE', *, *, #14051, .F. ) ;
#13942=VERTEX_POINT ( 'NONE', #12535 ) ;
#13943=ORIENTED_EDGE ( 'NONE', *, *, #14156, .T. ) ;
#13951=AXIS2_PLACEMENT_3D ( 'NONE', #6305, #8868, #3804 ) ;
#13970=DIRECTION ( 'NONE',  ( 0.000000000000000000, -0.000000000000000000, 1.000000000000000000 ) ) ;
#13997=CARTESIAN_POINT ( 'NONE',  ( 2.500000000000000000, 217.0000000000000284, -44.93050188902856945 ) ) ;
#14011=CARTESIAN_POINT ( 'NONE',  ( 43.87482193696061472, 267.0000000000000000, -10.00000000000000178 ) ) ;
#14041=DIRECTION ( 'NONE',  ( 0.000000000000000000, 1.000000000000000000, -0.000000000000000000 ) ) ;
#14051=EDGE_CURVE ( 'NONE', #9545, #2064, #13802, .T. ) ;
#14053=CARTESIAN_POINT ( 'NONE',  ( 47.28673853953970507, 260.3313524089090265, 10.00000000000000178 ) ) ;
#14100=CARTESIAN_POINT ( 'NONE',  ( 2.499999999999999556, 247.0000000000000568, -49.17157287525380127 ) ) ;
#14122=EDGE_CURVE ( 'NONE', #3157, #9937, #696, .T. ) ;
#14130=CARTESIAN_POINT ( 'NONE',  ( 43.87482193696061472, 257.0000000000001137, -10.00000000000000000 ) ) ;
#14143=CARTESIAN_POINT ( 'NONE',  ( -0.5000000000000000000, 245.0000000000000284, -49.99999999999999289 ) ) ;
#14144=MANIFOLD_SOLID_BREP ( 'Cut-Extrude1', #4698 ) ;
#14156=EDGE_CURVE ( 'NONE', #3758, #13942, #14493, .T. ) ;
#14163=DIRECTION ( 'NONE',  ( -0.000000000000000000, 1.000000000000000000, -0.000000000000000000 ) ) ;
#14189=CARTESIAN_POINT ( 'NONE',  ( -48.98979485566356828, 261.9999999999999432, -9.999999999999994671 ) ) ;
#14191=ORIENTED_EDGE ( 'NONE', *, *, #6967, .T. ) ;
#14257=ORIENTED_EDGE ( 'NONE', *, *, #13422, .F. ) ;
#14268=CARTESIAN_POINT ( 'NONE',  ( 5.510910596163089556E-15, 267.0000000000000000, -45.00000000000000000 ) ) ;
#14271=VERTEX_POINT ( 'NONE', #2990 ) ;
#14280=CARTESIAN_POINT ( 'NONE',  ( -0.5000000000000000000, 242.0000000000000284, 49.99999999999999289 ) ) ;
#14298=VECTOR ( 'NONE', #3060, 1000.000000000000000 ) ;
#14302=DIRECTION ( 'NONE',  ( 0.000000000000000000, 0.000000000000000000, 1.000000000000000000 ) ) ;
#14306=EDGE_CURVE ( 'NONE', #1328, #4312, #12554, .T. ) ;
#14309=CARTESIAN_POINT ( 'NONE',  ( 2.500000000000000000, 242.0000000000000284, 47.99999999999999289 ) ) ;
#14316=FACE_OUTER_BOUND ( 'NONE', #5228, .T. ) ;
#14317=VERTEX_POINT ( 'NONE', #4329 ) ;
#14321=PLANE ( 'NONE',  #12655 ) ;
#14344=DIRECTION ( 'NONE',  ( 0.000000000000000000, 0.000000000000000000, 1.000000000000000000 ) ) ;
#14353=ORIENTED_EDGE ( 'NONE', *, *, #8383, .T. ) ;
#14368=CARTESIAN_POINT ( 'NONE',  ( -45.00000000000000000, 262.0000000000000000, -10.00000000000000178 ) ) ;
#14374=EDGE_LOOP ( 'NONE', ( #6912, #8623, #12833, #9400, #10657 ) ) ;
#14441=LINE ( 'NONE', #14368, #7368 ) ;
#14464=ORIENTED_EDGE ( 'NONE', *, *, #826, .F. ) ;
#14470=FACE_OUTER_BOUND ( 'NONE', #3548, .T. ) ;
#14478=AXIS2_PLACEMENT_3D ( 'NONE', #15771, #9383, #5577 ) ;
#14493=CIRCLE ( 'NONE', #7358, 45.00000000000000000 ) ;
#14494=AXIS2_PLACEMENT_3D ( 'NONE', #8995, #16397, #7742 ) ;
#14589=VERTEX_POINT ( 'NONE', #13936 ) ;
#14593=CONICAL_SURFACE ( 'NONE', #2307, 49.99999999999999289, 0.7853981633974642662 ) ;
#14607=ADVANCED_FACE ( 'NONE', ( #15107 ), #3567, .F. ) ;
#14616=EDGE_LOOP ( 'NONE', ( #3618, #7421, #10635, #15502 ) ) ;
#14625=DIRECTION ( 'NONE',  ( 0.000000000000000000, 1.000000000000000000, 0.000000000000000000 ) ) ;
#14640=DIRECTION ( 'NONE',  ( 1.000000000000000000, -0.000000000000000000, 0.000000000000000000 ) ) ;
#14645=CARTESIAN_POINT ( 'NONE',  ( -2.499999999999999556, 242.0000000000000853, -49.17157287525380127 ) ) ;
#14664=CARTESIAN_POINT ( 'NONE',  ( -45.00000000000000000, 262.0000000000000000, 0.000000000000000000 ) ) ;
#14677=CARTESIAN_POINT ( 'NONE',  ( 2.500000000000000000, 247.0000000000000284, -47.99999999999999289 ) ) ;
#14680=CARTESIAN_POINT ( 'NONE',  ( -2.499999999999999556, 247.0000000000000568, 49.17157287525380127 ) ) ;
#14690=VERTEX_POINT ( 'NONE', #2801 ) ;
#14700=DIRECTION ( 'NONE',  ( 1.000000000000000000, 0.000000000000000000, -0.000000000000000000 ) ) ;
#14714=ORIENTED_EDGE ( 'NONE', *, *, #11120, .T. ) ;
#14715=CARTESIAN_POINT ( 'NONE',  ( 0.000000000000000000, 262.0000000000000000, 0.000000000000000000 ) ) ;
#14753=AXIS2_PLACEMENT_3D ( 'NONE', #3927, #11731, #1256 ) ;
#14789=DIRECTION ( 'NONE',  ( 0.000000000000000000, 0.000000000000000000, 1.000000000000000000 ) ) ;
#14808=DIRECTION ( 'NONE',  ( 0.000000000000000000, 0.000000000000000000, -1.000000000000000000 ) ) ;
#14842=ORIENTED_EDGE ( 'NONE', *, *, #15660, .T. ) ;
#14849=DIRECTION ( 'NONE',  ( -1.000000000000000000, 0.000000000000000000, -0.000000000000000000 ) ) ;
#14880=FACE_OUTER_BOUND ( 'NONE', #14374, .T. ) ;
#14884=ADVANCED_FACE ( 'NONE', ( #15931 ), #4635, .F. ) ;
#14885=DIRECTION ( 'NONE',  ( -0.000000000000000000, 1.000000000000000000, -0.000000000000000000 ) ) ;
#14921=ORIENTED_EDGE ( 'NONE', *, *, #13728, .F. ) ;
#14950=DIRECTION ( 'NONE',  ( 0.000000000000000000, -1.000000000000000000, 0.000000000000000000 ) ) ;
#14991=ORIENTED_EDGE ( 'NONE', *, *, #11036, .T. ) ;
#15008=CONICAL_SURFACE ( 'NONE', #9188, 49.99999999999999289, 0.7853981633974642662 ) ;
#15013=LINE ( 'NONE', #2054, #9454 ) ;
#15018=DIRECTION ( 'NONE',  ( -1.000000000000000000, 0.000000000000000000, 0.000000000000000000 ) ) ;
#15041=CARTESIAN_POINT ( 'NONE',  ( 2.499999999999999556, 247.0000000000000568, 49.17157287525380127 ) ) ;
#15062=CARTESIAN_POINT ( 'NONE',  ( 0.000000000000000000, 262.0000000000000000, 0.000000000000000000 ) ) ;
#15077=EDGE_LOOP ( 'NONE', ( #7844, #16039, #6013, #814 ) ) ;
#15106=CARTESIAN_POINT ( 'NONE',  ( 2.500000000000000000, 247.0000000000000284, -40.00000000000000000 ) ) ;
#15107=FACE_OUTER_BOUND ( 'NONE', #12026, .T. ) ;
#15127=DIRECTION ( 'NONE',  ( -1.000000000000000000, 0.000000000000000000, 0.000000000000000000 ) ) ;
#15145=ADVANCED_FACE ( 'NONE', ( #14316 ), #2935, .T. ) ;
#15157=DIRECTION ( 'NONE',  ( 0.000000000000000000, 0.000000000000000000, -1.000000000000000000 ) ) ;
#15195=PLANE ( 'NONE',  #11941 ) ;
#15197=DIRECTION ( 'NONE',  ( -1.000000000000000000, 0.000000000000000000, 0.000000000000000000 ) ) ;
#15200=CARTESIAN_POINT ( 'NONE',  ( -43.87482193696061472, 267.0000000000000000, 10.00000000000000178 ) ) ;
#15222=PLANE ( 'NONE',  #16110 ) ;
#15226=EDGE_CURVE ( 'NONE', #9638, #14271, #7010, .T. ) ;
#15236=DIRECTION ( 'NONE',  ( -0.000000000000000000, -1.000000000000000000, -0.000000000000000000 ) ) ;
#15239=VECTOR ( 'NONE', #11685, 1000.000000000000000 ) ;
#15275=CARTESIAN_POINT ( 'NONE',  ( 43.87482193696061472, 257.0000000000001137, -10.00000000000000000 ) ) ;
#15293=SURFACE_STYLE_FILL_AREA ( #11554 ) ;
#15301=CARTESIAN_POINT ( 'NONE',  ( 43.87482193696061472, 257.0000000000001137, 10.00000000000000178 ) ) ;
#15305=FACE_OUTER_BOUND ( 'NONE', #8309, .T. ) ;
#15306=CARTESIAN_POINT ( 'NONE',  ( 0.000000000000000000, 217.0000000000000284, 45.00000000000000000 ) ) ;
#15347=FACE_OUTER_BOUND ( 'NONE', #12606, .T. ) ;
#15363=ORIENTED_EDGE ( 'NONE', *, *, #8269, .T. ) ;
#15415=CARTESIAN_POINT ( 'NONE',  ( 5.510910596163089556E-15, 217.0000000000000284, -45.00000000000000000 ) ) ;
#15423=VERTEX_POINT ( 'NONE', #15306 ) ;
#15467=DIRECTION ( 'NONE',  ( 1.000000000000000000, 0.000000000000000000, 0.000000000000000000 ) ) ;
#15502=ORIENTED_EDGE ( 'NONE', *, *, #590, .T. ) ;
#15562=DIRECTION ( 'NONE',  ( 0.000000000000000000, 1.000000000000000000, 0.000000000000000000 ) ) ;
#15571=ORIENTED_EDGE ( 'NONE', *, *, #13920, .F. ) ;
#15575=DIRECTION ( 'NONE',  ( 0.000000000000000000, 0.000000000000000000, 1.000000000000000000 ) ) ;
#15578=VECTOR ( 'NONE', #3309, 1000.000000000000000 ) ;
#15599=CARTESIAN_POINT ( 'NONE',  ( 2.500000000000000000, 242.0000000000000284, 44.93050188902856945 ) ) ;
#15611=ORIENTED_EDGE ( 'NONE', *, *, #15955, .T. ) ;
#15620=CARTESIAN_POINT ( 'NONE',  ( 4.898587196589413026E-15, 267.0000000000000000, -40.00000000000000000 ) ) ;
#15633=AXIS2_PLACEMENT_3D ( 'NONE', #11880, #314, #9232 ) ;
#15655=PLANE ( 'NONE',  #6030 ) ;
#15660=EDGE_CURVE ( 'NONE', #9638, #2476, #9376, .T. ) ;
#15671=LINE ( 'NONE', #4294, #9415 ) ;
#15686=ORIENTED_EDGE ( 'NONE', *, *, #590, .F. ) ;
#15707=DIRECTION ( 'NONE',  ( 0.000000000000000000, -1.000000000000000000, 0.000000000000000000 ) ) ;
#15712=CARTESIAN_POINT ( 'NONE',  ( 0.000000000000000000, 267.0000000000000000, 40.00000000000000000 ) ) ;
#15743=EDGE_CURVE ( 'NONE', #14271, #9033, #5835, .T. ) ;
#15747=CIRCLE ( 'NONE', #3069, 45.00000000000000000 ) ;
#15768=CYLINDRICAL_SURFACE ( 'NONE', #16391, 2.000000000000001776 ) ;
#15771=CARTESIAN_POINT ( 'NONE',  ( 0.000000000000000000, 217.0000000000000284, 0.000000000000000000 ) ) ;
#15812=AXIS2_PLACEMENT_3D ( 'NONE', #2158, #11073, #8560 ) ;
#15824=CIRCLE ( 'NONE', #8657, 49.99999999999999289 ) ;
#15828=( GEOMETRIC_REPRESENTATION_CONTEXT ( 3 ) GLOBAL_UNCERTAINTY_ASSIGNED_CONTEXT ( ( #10262 ) ) GLOBAL_UNIT_ASSIGNED_CONTEXT ( ( #1216, #49, #129 ) ) REPRESENTATION_CONTEXT ( 'NONE', 'WORKASPACE' ) );
#15831=EDGE_CURVE ( 'NONE', #5700, #14317, #7244, .T. ) ;
#15858=EDGE_CURVE ( 'NONE', #7640, #14690, #1943, .T. ) ;
#15891=CARTESIAN_POINT ( 'NONE',  ( 0.000000000000000000, 261.9999999999999432, 0.000000000000000000 ) ) ;
#15903=CARTESIAN_POINT ( 'NONE',  ( -2.500000000000000000, 244.0000000000000284, 47.99999999999999289 ) ) ;
#15906=FACE_OUTER_BOUND ( 'NONE', #8932, .T. ) ;
#15914=EDGE_CURVE ( 'NONE', #5468, #4312, #12637, .T. ) ;
#15931=FACE_OUTER_BOUND ( 'NONE', #10056, .T. ) ;
#15932=EDGE_LOOP ( 'NONE', ( #8175, #10650, #6716, #14714 ) ) ;
#15949=CARTESIAN_POINT ( 'NONE',  ( 0.000000000000000000, 261.9999999999999432, 0.000000000000000000 ) ) ;
#15955=EDGE_CURVE ( 'NONE', #6571, #14589, #5015, .T. ) ;
#15963=DIRECTION ( 'NONE',  ( 0.000000000000000000, 0.000000000000000000, 1.000000000000000000 ) ) ;
#15965=CARTESIAN_POINT ( 'NONE',  ( 5.510910596163089556E-15, 242.0000000000000284, -45.00000000000000000 ) ) ;
#16039=ORIENTED_EDGE ( 'NONE', *, *, #5916, .F. ) ;
#16059=CARTESIAN_POINT ( 'NONE',  ( 5.510910596163089556E-15, 257.0000000000001137, -45.00000000000000000 ) ) ;
#16074=CIRCLE ( 'NONE', #9967, 45.00000000000000000 ) ;
#16110=AXIS2_PLACEMENT_3D ( 'NONE', #5042, #2600, #1176 ) ;
#16141=DIRECTION ( 'NONE',  ( 0.000000000000000000, 0.000000000000000000, -1.000000000000000000 ) ) ;
#16151=ORIENTED_EDGE ( 'NONE', *, *, #2274, .T. ) ;
#16185=ORIENTED_EDGE ( 'NONE', *, *, #12934, .F. ) ;
#16213=LINE ( 'NONE', #2154, #7063 ) ;
#16232=PLANE ( 'NONE',  #11837 ) ;
#16264=VERTEX_POINT ( 'NONE', #14309 ) ;
#16266=CYLINDRICAL_SURFACE ( 'NONE', #121, 2.000000000000001776 ) ;
#16326=AXIS2_PLACEMENT_3D ( 'NONE', #3496, #8633, #7237 ) ;
#16342=ORIENTED_EDGE ( 'NONE', *, *, #7778, .F. ) ;
#16381=CARTESIAN_POINT ( 'NONE',  ( 4.898587196589413026E-15, 217.0000000000000284, -40.00000000000000000 ) ) ;
#16391=AXIS2_PLACEMENT_3D ( 'NONE', #4237, #11710, #4315 ) ;
#16393=ORIENTED_EDGE ( 'NONE', *, *, #14306, .F. ) ;
#16397=DIRECTION ( 'NONE',  ( 0.000000000000000000, 1.000000000000000000, 0.000000000000000000 ) ) ;
#16426=EDGE_CURVE ( 'NONE', #5700, #1977, #15747, .T. ) ;
#16435=ORIENTED_EDGE ( 'NONE', *, *, #8796, .F. ) ;
#16436=VERTEX_POINT ( 'NONE', #751 ) ;
#16444=( NAMED_UNIT ( * ) SI_UNIT ( $, .STERADIAN. ) SOLID_ANGLE_UNIT ( ) );
#16454=VECTOR ( 'NONE', #5807, 1000.000000000000000 ) ;
ENDSEC;
END-ISO-10303-21;
